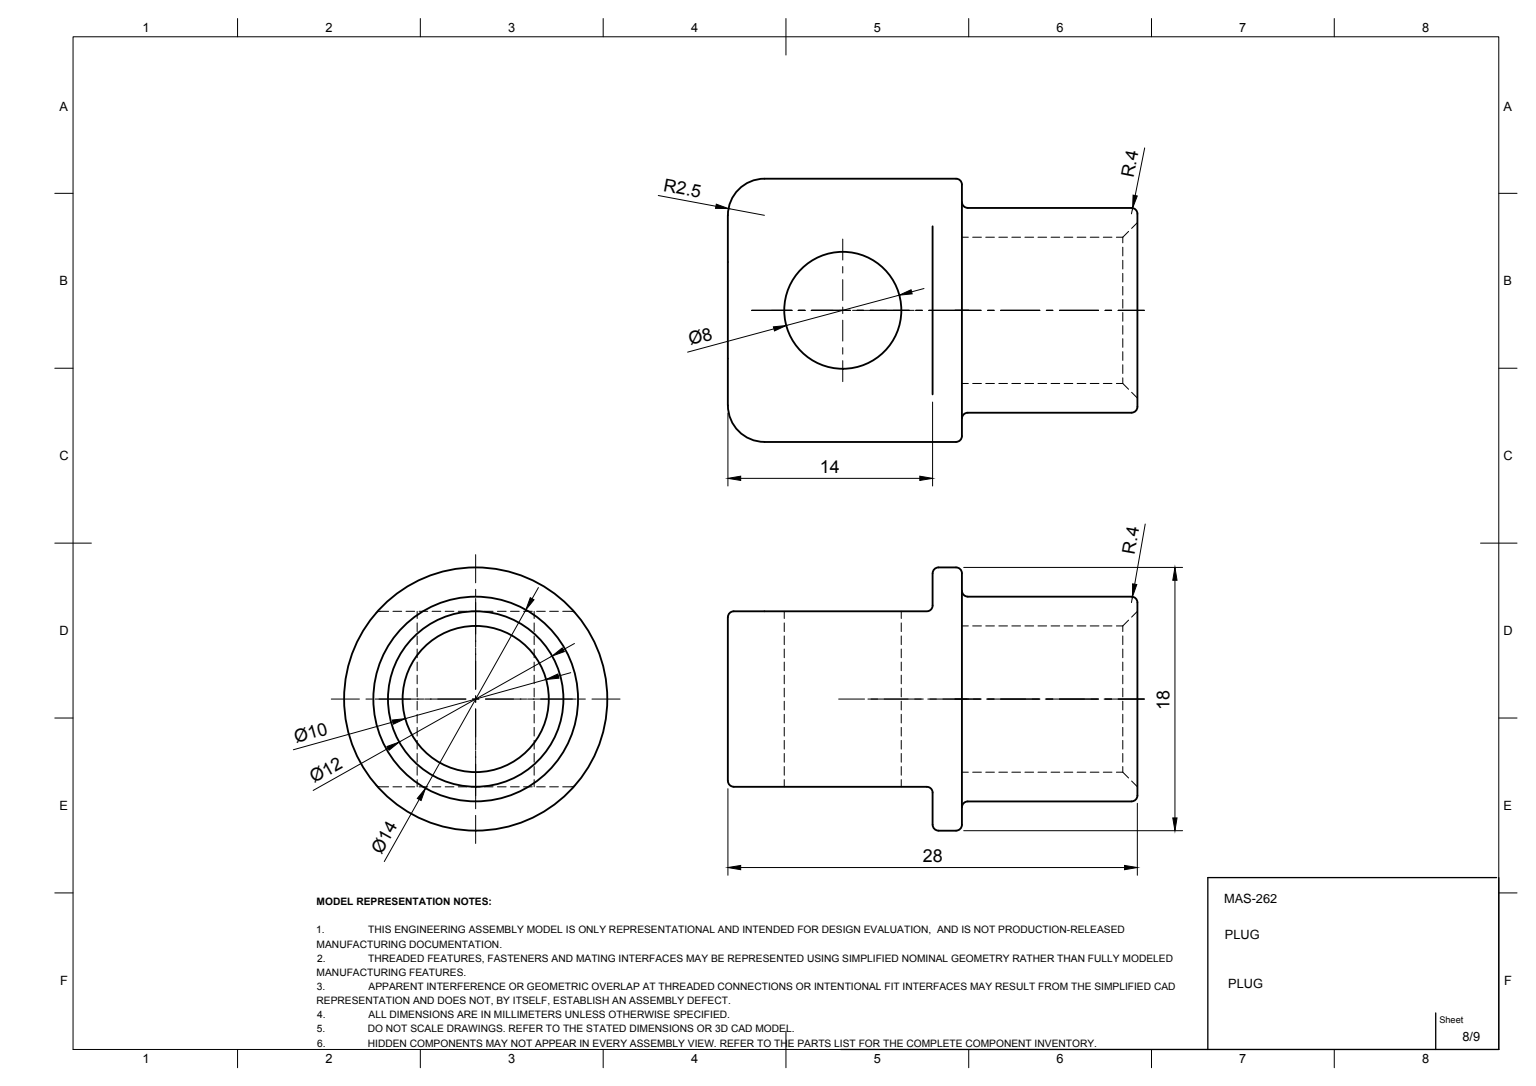
ISO-10303-21;
HEADER;
/* Generated by software containing ST-Developer
 * from STEP Tools, Inc. (www.steptools.com) 
 */

FILE_DESCRIPTION(
/* description */ (''),
/* implementation_level */ '2;1');

FILE_NAME(
/* name */ 'PLUG.step',
/* time_stamp */ '2026-10-07T02:13:48+06:00',
/* author */ (''),
/* organization */ (''),
/* preprocessor_version */ 'ST-DEVELOPER v20.2',
/* originating_system */ 'Autodesk Translation Framework v15.15.0.0',
/* authorisation */ '');

FILE_SCHEMA (('AUTOMOTIVE_DESIGN { 1 0 10303 214 3 1 1 }'));
ENDSEC;

DATA;
#10=MECHANICAL_DESIGN_GEOMETRIC_PRESENTATION_REPRESENTATION('',(#119),#17042);
#61=CONICAL_SURFACE('',#8902,5.5,0.785398163397441);
#76=B_SPLINE_SURFACE_WITH_KNOTS('',3,3,((#13698,#13699,#13700,#13701,#13702,
#13703),(#13704,#13705,#13706,#13707,#13708,#13709),(#13710,#13711,#13712,
#13713,#13714,#13715),(#13716,#13717,#13718,#13719,#13720,#13721),(#13722,
#13723,#13724,#13725,#13726,#13727)),.UNSPECIFIED.,.F.,.F.,.F.,(4,1,4),
(4,1,1,4),(0.,0.5,1.),(0.,0.0435664957825988,0.0599039317010734,0.0762413676195479),
 .UNSPECIFIED.);
#77=B_SPLINE_SURFACE_WITH_KNOTS('',3,3,((#13746,#13747,#13748,#13749,#13750,
#13751),(#13752,#13753,#13754,#13755,#13756,#13757),(#13758,#13759,#13760,
#13761,#13762,#13763),(#13764,#13765,#13766,#13767,#13768,#13769),(#13770,
#13771,#13772,#13773,#13774,#13775)),.UNSPECIFIED.,.F.,.F.,.F.,(4,1,4),
(4,1,1,4),(0.,0.5,1.),(0.,0.0163372895861103,0.0326745791722206,0.0762406847351813),
 .UNSPECIFIED.);
#78=B_SPLINE_SURFACE_WITH_KNOTS('',3,3,((#13800,#13801,#13802,#13803,#13804,
#13805),(#13806,#13807,#13808,#13809,#13810,#13811),(#13812,#13813,#13814,
#13815,#13816,#13817),(#13818,#13819,#13820,#13821,#13822,#13823),(#13824,
#13825,#13826,#13827,#13828,#13829)),.UNSPECIFIED.,.F.,.F.,.F.,(4,1,4),
(4,1,1,4),(0.,0.5,1.),(3.96177645312185E-16,0.061147749085529,0.0917216236282934,
0.214017121799351),.UNSPECIFIED.);
#79=B_SPLINE_SURFACE_WITH_KNOTS('',3,3,((#13851,#13852,#13853,#13854,#13855,
#13856),(#13857,#13858,#13859,#13860,#13861,#13862),(#13863,#13864,#13865,
#13866,#13867,#13868),(#13869,#13870,#13871,#13872,#13873,#13874),(#13875,
#13876,#13877,#13878,#13879,#13880)),.UNSPECIFIED.,.F.,.F.,.F.,(4,1,4),
(4,1,1,4),(0.,0.5,1.),(2.01858731750029E-18,0.0917257862177262,0.152876310362877,
0.214026834508028),.UNSPECIFIED.);
#80=B_SPLINE_SURFACE_WITH_KNOTS('',3,3,((#13926,#13927,#13928,#13929,#13930,
#13931),(#13932,#13933,#13934,#13935,#13936,#13937),(#13938,#13939,#13940,
#13941,#13942,#13943),(#13944,#13945,#13946,#13947,#13948,#13949),(#13950,
#13951,#13952,#13953,#13954,#13955)),.UNSPECIFIED.,.F.,.F.,.F.,(4,1,4),
(4,1,1,4),(0.,0.5,1.),(0.,0.0163372896496662,0.0326745792993324,0.0762406850317755),
 .UNSPECIFIED.);
#81=B_SPLINE_SURFACE_WITH_KNOTS('',3,3,((#13974,#13975,#13976,#13977,#13978,
#13979),(#13980,#13981,#13982,#13983,#13984,#13985),(#13986,#13987,#13988,
#13989,#13990,#13991),(#13992,#13993,#13994,#13995,#13996,#13997),(#13998,
#13999,#14000,#14001,#14002,#14003)),.UNSPECIFIED.,.F.,.F.,.F.,(4,1,4),
(4,1,1,4),(0.,0.5,1.),(7.01665201425609E-18,0.0435664948259872,0.0599039303857324,
0.0762413659454776),.UNSPECIFIED.);
#82=B_SPLINE_SURFACE_WITH_KNOTS('',3,3,((#14027,#14028,#14029,#14030,#14031,
#14032),(#14033,#14034,#14035,#14036,#14037,#14038),(#14039,#14040,#14041,
#14042,#14043,#14044),(#14045,#14046,#14047,#14048,#14049,#14050),(#14051,
#14052,#14053,#14054,#14055,#14056)),.UNSPECIFIED.,.F.,.F.,.F.,(4,1,4),
(4,1,1,4),(0.,0.5,1.),(6.74145042959343E-15,0.0611477488274177,0.0917216232411232,
0.214017120895945),.UNSPECIFIED.);
#83=B_SPLINE_SURFACE_WITH_KNOTS('',3,3,((#14069,#14070,#14071,#14072,#14073,
#14074),(#14075,#14076,#14077,#14078,#14079,#14080),(#14081,#14082,#14083,
#14084,#14085,#14086),(#14087,#14088,#14089,#14090,#14091,#14092),(#14093,
#14094,#14095,#14096,#14097,#14098)),.UNSPECIFIED.,.F.,.F.,.F.,(4,1,4),
(4,1,1,4),(0.,0.5,1.),(0.,0.0917257862177262,0.152876310362877,0.214026834508028),
 .UNSPECIFIED.);
#95=SHAPE_REPRESENTATION_RELATIONSHIP('SRR','None',#17091,#107);
#107=ADVANCED_BREP_SHAPE_REPRESENTATION('',(#131),#17035);
#119=STYLED_ITEM('',(#17154),#131);
#131=MANIFOLD_SOLID_BREP('Body1',#8120);
#164=FACE_BOUND('',#1281,.T.);
#165=FACE_BOUND('',#1294,.T.);
#166=FACE_BOUND('',#1299,.T.);
#167=FACE_BOUND('',#1304,.T.);
#226=TOROIDAL_SURFACE('',#8852,8.6,0.4);
#227=TOROIDAL_SURFACE('',#8859,6.5,2.5);
#228=TOROIDAL_SURFACE('',#8875,8.6,0.4);
#229=TOROIDAL_SURFACE('',#8885,6.5,2.5);
#230=TOROIDAL_SURFACE('',#8886,8.6,0.4);
#231=TOROIDAL_SURFACE('',#8891,7.4,0.4);
#232=TOROIDAL_SURFACE('',#8897,6.6,0.4);
#394=PLANE('',#8856);
#395=PLANE('',#8861);
#396=PLANE('',#8863);
#397=PLANE('',#8882);
#398=PLANE('',#8884);
#399=PLANE('',#8889);
#400=PLANE('',#8900);
#401=PLANE('',#8907);
#766=FACE_OUTER_BOUND('',#1269,.T.);
#767=FACE_OUTER_BOUND('',#1270,.T.);
#768=FACE_OUTER_BOUND('',#1271,.T.);
#769=FACE_OUTER_BOUND('',#1272,.T.);
#770=FACE_OUTER_BOUND('',#1273,.T.);
#771=FACE_OUTER_BOUND('',#1274,.T.);
#772=FACE_OUTER_BOUND('',#1275,.T.);
#773=FACE_OUTER_BOUND('',#1276,.T.);
#774=FACE_OUTER_BOUND('',#1277,.T.);
#775=FACE_OUTER_BOUND('',#1278,.T.);
#776=FACE_OUTER_BOUND('',#1279,.T.);
#777=FACE_OUTER_BOUND('',#1280,.T.);
#778=FACE_OUTER_BOUND('',#1282,.T.);
#779=FACE_OUTER_BOUND('',#1283,.T.);
#780=FACE_OUTER_BOUND('',#1284,.T.);
#781=FACE_OUTER_BOUND('',#1285,.T.);
#782=FACE_OUTER_BOUND('',#1286,.T.);
#783=FACE_OUTER_BOUND('',#1287,.T.);
#784=FACE_OUTER_BOUND('',#1288,.T.);
#785=FACE_OUTER_BOUND('',#1289,.T.);
#786=FACE_OUTER_BOUND('',#1290,.T.);
#787=FACE_OUTER_BOUND('',#1291,.T.);
#788=FACE_OUTER_BOUND('',#1292,.T.);
#789=FACE_OUTER_BOUND('',#1293,.T.);
#790=FACE_OUTER_BOUND('',#1295,.T.);
#791=FACE_OUTER_BOUND('',#1296,.T.);
#792=FACE_OUTER_BOUND('',#1297,.T.);
#793=FACE_OUTER_BOUND('',#1298,.T.);
#794=FACE_OUTER_BOUND('',#1300,.T.);
#795=FACE_OUTER_BOUND('',#1301,.T.);
#796=FACE_OUTER_BOUND('',#1302,.T.);
#797=FACE_OUTER_BOUND('',#1303,.T.);
#798=FACE_OUTER_BOUND('',#1305,.T.);
#799=FACE_OUTER_BOUND('',#1306,.T.);
#800=FACE_OUTER_BOUND('',#1307,.T.);
#801=FACE_OUTER_BOUND('',#1308,.T.);
#1269=EDGE_LOOP('',(#6539,#6540,#6541,#6542));
#1270=EDGE_LOOP('',(#6543,#6544,#6545,#6546));
#1271=EDGE_LOOP('',(#6547,#6548,#6549,#6550));
#1272=EDGE_LOOP('',(#6551,#6552,#6553,#6554));
#1273=EDGE_LOOP('',(#6555,#6556,#6557,#6558));
#1274=EDGE_LOOP('',(#6559,#6560,#6561,#6562));
#1275=EDGE_LOOP('',(#6563,#6564,#6565,#6566));
#1276=EDGE_LOOP('',(#6567,#6568,#6569,#6570));
#1277=EDGE_LOOP('',(#6571,#6572,#6573,#6574,#6575));
#1278=EDGE_LOOP('',(#6576,#6577,#6578,#6579));
#1279=EDGE_LOOP('',(#6580,#6581,#6582,#6583));
#1280=EDGE_LOOP('',(#6584,#6585,#6586,#6587,#6588,#6589));
#1281=EDGE_LOOP('',(#6590));
#1282=EDGE_LOOP('',(#6591,#6592));
#1283=EDGE_LOOP('',(#6593,#6594,#6595,#6596));
#1284=EDGE_LOOP('',(#6597,#6598,#6599,#6600));
#1285=EDGE_LOOP('',(#6601,#6602,#6603,#6604));
#1286=EDGE_LOOP('',(#6605,#6606,#6607,#6608));
#1287=EDGE_LOOP('',(#6609,#6610,#6611,#6612));
#1288=EDGE_LOOP('',(#6613,#6614,#6615,#6616));
#1289=EDGE_LOOP('',(#6617,#6618,#6619,#6620));
#1290=EDGE_LOOP('',(#6621,#6622,#6623,#6624));
#1291=EDGE_LOOP('',(#6625,#6626,#6627,#6628));
#1292=EDGE_LOOP('',(#6629,#6630,#6631,#6632,#6633,#6634,#6635,#6636,#6637,
#6638,#6639,#6640,#6641,#6642,#6643,#6644));
#1293=EDGE_LOOP('',(#6645,#6646,#6647,#6648,#6649,#6650));
#1294=EDGE_LOOP('',(#6651));
#1295=EDGE_LOOP('',(#6652,#6653));
#1296=EDGE_LOOP('',(#6654,#6655,#6656,#6657));
#1297=EDGE_LOOP('',(#6658,#6659,#6660,#6661));
#1298=EDGE_LOOP('',(#6662));
#1299=EDGE_LOOP('',(#6663));
#1300=EDGE_LOOP('',(#6664,#6665,#6666,#6667));
#1301=EDGE_LOOP('',(#6668,#6669,#6670,#6671,#6672));
#1302=EDGE_LOOP('',(#6673,#6674,#6675,#6676,#6677));
#1303=EDGE_LOOP('',(#6678));
#1304=EDGE_LOOP('',(#6679));
#1305=EDGE_LOOP('',(#6680,#6681,#6682,#6683));
#1306=EDGE_LOOP('',(#6684,#6685,#6686,#6687));
#1307=EDGE_LOOP('',(#6688,#6689,#6690,#6691));
#1308=EDGE_LOOP('',(#6692));
#1770=CIRCLE('',#8840,0.400000000000001);
#1771=CIRCLE('',#8841,0.399999999999991);
#1772=CIRCLE('',#8842,0.4);
#1773=CIRCLE('',#8843,0.400000000000001);
#1774=CIRCLE('',#8845,0.400000000000003);
#1775=CIRCLE('',#8846,0.4);
#1776=CIRCLE('',#8848,0.4);
#1777=CIRCLE('',#8849,0.4);
#1778=CIRCLE('',#8853,9.);
#1779=CIRCLE('',#8854,9.);
#1780=CIRCLE('',#8855,8.6);
#1781=CIRCLE('',#8857,6.5);
#1782=CIRCLE('',#8858,6.5);
#1783=CIRCLE('',#8860,9.);
#1784=CIRCLE('',#8862,4.);
#1785=CIRCLE('',#8864,0.4);
#1786=CIRCLE('',#8865,0.400000000000001);
#1787=CIRCLE('',#8866,0.400000000000001);
#1788=CIRCLE('',#8867,0.399999999999991);
#1789=CIRCLE('',#8869,0.4);
#1790=CIRCLE('',#8870,0.4);
#1791=CIRCLE('',#8872,0.399999999999999);
#1792=CIRCLE('',#8873,0.4);
#1793=CIRCLE('',#8876,9.);
#1794=CIRCLE('',#8877,8.6);
#1795=CIRCLE('',#8880,9.);
#1796=CIRCLE('',#8881,9.);
#1797=CIRCLE('',#8883,4.);
#1798=CIRCLE('',#8887,0.4);
#1799=CIRCLE('',#8888,8.6);
#1800=CIRCLE('',#8890,7.4);
#1801=CIRCLE('',#8892,7.);
#1802=CIRCLE('',#8893,0.4);
#1803=CIRCLE('',#8895,7.);
#1804=CIRCLE('',#8896,7.);
#1805=CIRCLE('',#8898,6.6);
#1806=CIRCLE('',#8899,0.4);
#1807=CIRCLE('',#8901,6.);
#1808=CIRCLE('',#8903,5.);
#1809=CIRCLE('',#8905,5.);
#1960=B_SPLINE_CURVE_WITH_KNOTS('',3,(#13730,#13731,#13732,#13733,#13734,
#13735),.UNSPECIFIED.,.F.,.F.,(4,1,1,4),(0.,0.0435664957825988,0.0599039317010734,
0.0762413676195479),.UNSPECIFIED.);
#1961=B_SPLINE_CURVE_WITH_KNOTS('',3,(#13739,#13740,#13741,#13742,#13743,
#13744),.UNSPECIFIED.,.F.,.F.,(4,1,1,4),(-0.0762413676195479,-0.0599039317010734,
-0.0435664957825988,0.),.UNSPECIFIED.);
#1962=B_SPLINE_CURVE_WITH_KNOTS('',3,(#13778,#13779,#13780,#13781,#13782,
#13783),.UNSPECIFIED.,.F.,.F.,(4,1,1,4),(-0.0762406847351813,-0.0326745791722206,
-0.0163372895861103,0.),.UNSPECIFIED.);
#1963=B_SPLINE_CURVE_WITH_KNOTS('',3,(#13787,#13788,#13789,#13790,#13791,
#13792),.UNSPECIFIED.,.F.,.F.,(4,1,1,4),(0.,0.0163372895861103,0.0326745791722206,
0.0762406847351813),.UNSPECIFIED.);
#1964=B_SPLINE_CURVE_WITH_KNOTS('',3,(#13833,#13834,#13835,#13836,#13837,
#13838),.UNSPECIFIED.,.F.,.F.,(4,1,1,4),(-0.214017121799351,-0.0917216236282934,
-0.061147749085529,-3.96177645312185E-16),.UNSPECIFIED.);
#1965=B_SPLINE_CURVE_WITH_KNOTS('',3,(#13839,#13840,#13841,#13842,#13843,
#13844),.UNSPECIFIED.,.F.,.F.,(4,1,1,4),(3.96177645312185E-16,0.061147749085529,
0.0917216236282934,0.214017121799351),.UNSPECIFIED.);
#1966=B_SPLINE_CURVE_WITH_KNOTS('',3,(#13884,#13885,#13886,#13887,#13888,
#13889),.UNSPECIFIED.,.F.,.F.,(4,1,1,4),(-0.214026834508028,-0.152876310362877,
-0.0917257862177262,-2.01858731750029E-18),.UNSPECIFIED.);
#1967=B_SPLINE_CURVE_WITH_KNOTS('',3,(#13890,#13891,#13892,#13893,#13894,
#13895),.UNSPECIFIED.,.F.,.F.,(4,1,1,4),(2.01858731750029E-18,0.0917257862177262,
0.152876310362877,0.214026834508028),.UNSPECIFIED.);
#1968=B_SPLINE_CURVE_WITH_KNOTS('',3,(#13916,#13917,#13918,#13919,#13920,
#13921),.UNSPECIFIED.,.F.,.F.,(4,1,1,4),(-0.214017120895945,-0.0917216232411232,
-0.0611477488274177,-6.74145042959343E-15),.UNSPECIFIED.);
#1969=B_SPLINE_CURVE_WITH_KNOTS('',3,(#13958,#13959,#13960,#13961,#13962,
#13963),.UNSPECIFIED.,.F.,.F.,(4,1,1,4),(-0.0762406850317755,-0.0326745792993324,
-0.0163372896496662,0.),.UNSPECIFIED.);
#1970=B_SPLINE_CURVE_WITH_KNOTS('',3,(#13967,#13968,#13969,#13970,#13971,
#13972),.UNSPECIFIED.,.F.,.F.,(4,1,1,4),(0.,0.0163372896496662,0.0326745792993324,
0.0762406850317755),.UNSPECIFIED.);
#1971=B_SPLINE_CURVE_WITH_KNOTS('',3,(#14006,#14007,#14008,#14009,#14010,
#14011),.UNSPECIFIED.,.F.,.F.,(4,1,1,4),(7.01665201425609E-18,0.0435664948259872,
0.0599039303857324,0.0762413659454776),.UNSPECIFIED.);
#1972=B_SPLINE_CURVE_WITH_KNOTS('',3,(#14015,#14016,#14017,#14018,#14019,
#14020),.UNSPECIFIED.,.F.,.F.,(4,1,1,4),(-0.0762413659454776,-0.0599039303857324,
-0.0435664948259872,-7.01665201425609E-18),.UNSPECIFIED.);
#1973=B_SPLINE_CURVE_WITH_KNOTS('',3,(#14059,#14060,#14061,#14062,#14063,
#14064),.UNSPECIFIED.,.F.,.F.,(4,1,1,4),(6.74145042959343E-15,0.0611477488274177,
0.0917216232411232,0.214017120895945),.UNSPECIFIED.);
#1974=B_SPLINE_CURVE_WITH_KNOTS('',3,(#14102,#14103,#14104,#14105,#14106,
#14107),.UNSPECIFIED.,.F.,.F.,(4,1,1,4),(-0.214026834508028,-0.152876310362877,
-0.0917257862177262,0.),.UNSPECIFIED.);
#1975=B_SPLINE_CURVE_WITH_KNOTS('',3,(#14108,#14109,#14110,#14111,#14112,
#14113),.UNSPECIFIED.,.F.,.F.,(4,1,1,4),(0.,0.0917257862177262,0.152876310362877,
0.214026834508028),.UNSPECIFIED.);
#2430=LINE('',#13798,#3008);
#2431=LINE('',#13799,#3009);
#2432=LINE('',#13849,#3010);
#2433=LINE('',#13850,#3011);
#2434=LINE('',#13897,#3012);
#2435=LINE('',#13898,#3013);
#2436=LINE('',#13900,#3014);
#2437=LINE('',#13901,#3015);
#2438=LINE('',#13911,#3016);
#2439=LINE('',#14025,#3017);
#2440=LINE('',#14026,#3018);
#2441=LINE('',#14068,#3019);
#2442=LINE('',#14115,#3020);
#2443=LINE('',#14116,#3021);
#2444=LINE('',#14121,#3022);
#2445=LINE('',#14122,#3023);
#2446=LINE('',#14126,#3024);
#2447=LINE('',#14148,#3025);
#2448=LINE('',#14159,#3026);
#2449=LINE('',#14163,#3027);
#2450=LINE('',#14166,#3028);
#3008=VECTOR('',#10831,20.);
#3009=VECTOR('',#10832,20.);
#3010=VECTOR('',#10839,20.);
#3011=VECTOR('',#10840,20.);
#3012=VECTOR('',#10845,20.);
#3013=VECTOR('',#10846,20.);
#3014=VECTOR('',#10849,20.);
#3015=VECTOR('',#10850,20.);
#3016=VECTOR('',#10863,20.);
#3017=VECTOR('',#10888,20.);
#3018=VECTOR('',#10889,20.);
#3019=VECTOR('',#10896,20.);
#3020=VECTOR('',#10901,20.);
#3021=VECTOR('',#10902,20.);
#3022=VECTOR('',#10911,20.);
#3023=VECTOR('',#10912,20.);
#3024=VECTOR('',#10917,9.);
#3025=VECTOR('',#10948,7.);
#3026=VECTOR('',#10963,5.5);
#3027=VECTOR('',#10968,5.);
#3028=VECTOR('',#10973,4.);
#3625=VERTEX_POINT('',#13728);
#3626=VERTEX_POINT('',#13729);
#3627=VERTEX_POINT('',#13736);
#3628=VERTEX_POINT('',#13738);
#3629=VERTEX_POINT('',#13776);
#3630=VERTEX_POINT('',#13777);
#3631=VERTEX_POINT('',#13784);
#3632=VERTEX_POINT('',#13786);
#3633=VERTEX_POINT('',#13795);
#3634=VERTEX_POINT('',#13796);
#3635=VERTEX_POINT('',#13830);
#3636=VERTEX_POINT('',#13831);
#3637=VERTEX_POINT('',#13846);
#3638=VERTEX_POINT('',#13847);
#3639=VERTEX_POINT('',#13881);
#3640=VERTEX_POINT('',#13882);
#3641=VERTEX_POINT('',#13903);
#3642=VERTEX_POINT('',#13908);
#3643=VERTEX_POINT('',#13910);
#3644=VERTEX_POINT('',#13914);
#3645=VERTEX_POINT('',#13923);
#3646=VERTEX_POINT('',#13956);
#3647=VERTEX_POINT('',#13957);
#3648=VERTEX_POINT('',#13964);
#3649=VERTEX_POINT('',#13966);
#3650=VERTEX_POINT('',#14004);
#3651=VERTEX_POINT('',#14005);
#3652=VERTEX_POINT('',#14012);
#3653=VERTEX_POINT('',#14014);
#3654=VERTEX_POINT('',#14023);
#3655=VERTEX_POINT('',#14057);
#3656=VERTEX_POINT('',#14066);
#3657=VERTEX_POINT('',#14099);
#3658=VERTEX_POINT('',#14100);
#3659=VERTEX_POINT('',#14125);
#3660=VERTEX_POINT('',#14129);
#3661=VERTEX_POINT('',#14134);
#3662=VERTEX_POINT('',#14138);
#3663=VERTEX_POINT('',#14141);
#3664=VERTEX_POINT('',#14145);
#3665=VERTEX_POINT('',#14146);
#3666=VERTEX_POINT('',#14151);
#3667=VERTEX_POINT('',#14155);
#3668=VERTEX_POINT('',#14158);
#3669=VERTEX_POINT('',#14162);
#4637=EDGE_CURVE('',#3625,#3626,#1960,.F.);
#4638=EDGE_CURVE('',#3627,#3625,#1770,.T.);
#4639=EDGE_CURVE('',#3627,#3628,#1961,.T.);
#4640=EDGE_CURVE('',#3626,#3628,#1771,.T.);
#4641=EDGE_CURVE('',#3629,#3630,#1962,.T.);
#4642=EDGE_CURVE('',#3631,#3630,#1772,.T.);
#4643=EDGE_CURVE('',#3632,#3631,#1963,.F.);
#4644=EDGE_CURVE('',#3629,#3632,#1773,.T.);
#4645=EDGE_CURVE('',#3633,#3634,#1774,.T.);
#4646=EDGE_CURVE('',#3634,#3627,#2430,.T.);
#4647=EDGE_CURVE('',#3625,#3633,#2431,.T.);
#4648=EDGE_CURVE('',#3635,#3636,#1775,.T.);
#4649=EDGE_CURVE('',#3636,#3634,#1964,.T.);
#4650=EDGE_CURVE('',#3633,#3635,#1965,.T.);
#4651=EDGE_CURVE('',#3637,#3638,#1776,.T.);
#4652=EDGE_CURVE('',#3638,#3636,#2432,.T.);
#4653=EDGE_CURVE('',#3635,#3637,#2433,.T.);
#4654=EDGE_CURVE('',#3639,#3640,#1777,.T.);
#4655=EDGE_CURVE('',#3640,#3638,#1966,.T.);
#4656=EDGE_CURVE('',#3637,#3639,#1967,.T.);
#4657=EDGE_CURVE('',#3630,#3640,#2434,.T.);
#4658=EDGE_CURVE('',#3639,#3631,#2435,.T.);
#4659=EDGE_CURVE('',#3631,#3625,#2436,.T.);
#4660=EDGE_CURVE('',#3626,#3632,#2437,.T.);
#4661=EDGE_CURVE('',#3628,#3641,#1778,.T.);
#4662=EDGE_CURVE('',#3641,#3629,#1779,.T.);
#4663=EDGE_CURVE('',#3632,#3626,#1780,.T.);
#4664=EDGE_CURVE('',#3642,#3638,#1781,.T.);
#4665=EDGE_CURVE('',#3643,#3642,#2438,.T.);
#4666=EDGE_CURVE('',#3636,#3643,#1782,.T.);
#4667=EDGE_CURVE('',#3640,#3644,#1783,.T.);
#4668=EDGE_CURVE('',#3642,#3644,#1968,.T.);
#4669=EDGE_CURVE('',#3645,#3645,#1784,.T.);
#4670=EDGE_CURVE('',#3646,#3647,#1969,.T.);
#4671=EDGE_CURVE('',#3648,#3647,#1785,.T.);
#4672=EDGE_CURVE('',#3649,#3648,#1970,.F.);
#4673=EDGE_CURVE('',#3646,#3649,#1786,.T.);
#4674=EDGE_CURVE('',#3650,#3651,#1971,.F.);
#4675=EDGE_CURVE('',#3652,#3650,#1787,.T.);
#4676=EDGE_CURVE('',#3652,#3653,#1972,.T.);
#4677=EDGE_CURVE('',#3651,#3653,#1788,.T.);
#4678=EDGE_CURVE('',#3654,#3644,#1789,.T.);
#4679=EDGE_CURVE('',#3644,#3652,#2439,.T.);
#4680=EDGE_CURVE('',#3650,#3654,#2440,.T.);
#4681=EDGE_CURVE('',#3655,#3642,#1790,.T.);
#4682=EDGE_CURVE('',#3654,#3655,#1973,.T.);
#4683=EDGE_CURVE('',#3656,#3643,#1791,.T.);
#4684=EDGE_CURVE('',#3655,#3656,#2441,.T.);
#4685=EDGE_CURVE('',#3657,#3658,#1792,.T.);
#4686=EDGE_CURVE('',#3658,#3643,#1974,.T.);
#4687=EDGE_CURVE('',#3656,#3657,#1975,.T.);
#4688=EDGE_CURVE('',#3647,#3658,#2442,.T.);
#4689=EDGE_CURVE('',#3657,#3648,#2443,.T.);
#4690=EDGE_CURVE('',#3653,#3646,#1793,.T.);
#4691=EDGE_CURVE('',#3649,#3651,#1794,.T.);
#4692=EDGE_CURVE('',#3648,#3650,#2444,.T.);
#4693=EDGE_CURVE('',#3651,#3649,#2445,.T.);
#4694=EDGE_CURVE('',#3658,#3634,#1795,.T.);
#4695=EDGE_CURVE('',#3641,#3659,#2446,.T.);
#4696=EDGE_CURVE('',#3659,#3659,#1796,.T.);
#4697=EDGE_CURVE('',#3660,#3660,#1797,.T.);
#4698=EDGE_CURVE('',#3659,#3661,#1798,.T.);
#4699=EDGE_CURVE('',#3661,#3661,#1799,.T.);
#4700=EDGE_CURVE('',#3662,#3662,#1800,.T.);
#4701=EDGE_CURVE('',#3663,#3663,#1801,.T.);
#4702=EDGE_CURVE('',#3663,#3662,#1802,.T.);
#4703=EDGE_CURVE('',#3664,#3665,#1803,.T.);
#4704=EDGE_CURVE('',#3664,#3663,#2447,.T.);
#4705=EDGE_CURVE('',#3665,#3664,#1804,.T.);
#4706=EDGE_CURVE('',#3666,#3666,#1805,.T.);
#4707=EDGE_CURVE('',#3666,#3665,#1806,.T.);
#4708=EDGE_CURVE('',#3667,#3667,#1807,.T.);
#4709=EDGE_CURVE('',#3667,#3668,#2448,.T.);
#4710=EDGE_CURVE('',#3668,#3668,#1808,.T.);
#4711=EDGE_CURVE('',#3668,#3669,#2449,.T.);
#4712=EDGE_CURVE('',#3669,#3669,#1809,.T.);
#4713=EDGE_CURVE('',#3645,#3660,#2450,.T.);
#6539=ORIENTED_EDGE('',*,*,#4637,.F.);
#6540=ORIENTED_EDGE('',*,*,#4638,.F.);
#6541=ORIENTED_EDGE('',*,*,#4639,.T.);
#6542=ORIENTED_EDGE('',*,*,#4640,.F.);
#6543=ORIENTED_EDGE('',*,*,#4641,.T.);
#6544=ORIENTED_EDGE('',*,*,#4642,.F.);
#6545=ORIENTED_EDGE('',*,*,#4643,.F.);
#6546=ORIENTED_EDGE('',*,*,#4644,.F.);
#6547=ORIENTED_EDGE('',*,*,#4645,.T.);
#6548=ORIENTED_EDGE('',*,*,#4646,.T.);
#6549=ORIENTED_EDGE('',*,*,#4638,.T.);
#6550=ORIENTED_EDGE('',*,*,#4647,.T.);
#6551=ORIENTED_EDGE('',*,*,#4648,.T.);
#6552=ORIENTED_EDGE('',*,*,#4649,.T.);
#6553=ORIENTED_EDGE('',*,*,#4645,.F.);
#6554=ORIENTED_EDGE('',*,*,#4650,.T.);
#6555=ORIENTED_EDGE('',*,*,#4651,.T.);
#6556=ORIENTED_EDGE('',*,*,#4652,.T.);
#6557=ORIENTED_EDGE('',*,*,#4648,.F.);
#6558=ORIENTED_EDGE('',*,*,#4653,.T.);
#6559=ORIENTED_EDGE('',*,*,#4654,.T.);
#6560=ORIENTED_EDGE('',*,*,#4655,.T.);
#6561=ORIENTED_EDGE('',*,*,#4651,.F.);
#6562=ORIENTED_EDGE('',*,*,#4656,.T.);
#6563=ORIENTED_EDGE('',*,*,#4642,.T.);
#6564=ORIENTED_EDGE('',*,*,#4657,.T.);
#6565=ORIENTED_EDGE('',*,*,#4654,.F.);
#6566=ORIENTED_EDGE('',*,*,#4658,.T.);
#6567=ORIENTED_EDGE('',*,*,#4643,.T.);
#6568=ORIENTED_EDGE('',*,*,#4659,.T.);
#6569=ORIENTED_EDGE('',*,*,#4637,.T.);
#6570=ORIENTED_EDGE('',*,*,#4660,.T.);
#6571=ORIENTED_EDGE('',*,*,#4640,.T.);
#6572=ORIENTED_EDGE('',*,*,#4661,.T.);
#6573=ORIENTED_EDGE('',*,*,#4662,.T.);
#6574=ORIENTED_EDGE('',*,*,#4644,.T.);
#6575=ORIENTED_EDGE('',*,*,#4663,.T.);
#6576=ORIENTED_EDGE('',*,*,#4652,.F.);
#6577=ORIENTED_EDGE('',*,*,#4664,.F.);
#6578=ORIENTED_EDGE('',*,*,#4665,.F.);
#6579=ORIENTED_EDGE('',*,*,#4666,.F.);
#6580=ORIENTED_EDGE('',*,*,#4655,.F.);
#6581=ORIENTED_EDGE('',*,*,#4667,.T.);
#6582=ORIENTED_EDGE('',*,*,#4668,.F.);
#6583=ORIENTED_EDGE('',*,*,#4664,.T.);
#6584=ORIENTED_EDGE('',*,*,#4647,.F.);
#6585=ORIENTED_EDGE('',*,*,#4659,.F.);
#6586=ORIENTED_EDGE('',*,*,#4658,.F.);
#6587=ORIENTED_EDGE('',*,*,#4656,.F.);
#6588=ORIENTED_EDGE('',*,*,#4653,.F.);
#6589=ORIENTED_EDGE('',*,*,#4650,.F.);
#6590=ORIENTED_EDGE('',*,*,#4669,.T.);
#6591=ORIENTED_EDGE('',*,*,#4660,.F.);
#6592=ORIENTED_EDGE('',*,*,#4663,.F.);
#6593=ORIENTED_EDGE('',*,*,#4670,.T.);
#6594=ORIENTED_EDGE('',*,*,#4671,.F.);
#6595=ORIENTED_EDGE('',*,*,#4672,.F.);
#6596=ORIENTED_EDGE('',*,*,#4673,.F.);
#6597=ORIENTED_EDGE('',*,*,#4674,.F.);
#6598=ORIENTED_EDGE('',*,*,#4675,.F.);
#6599=ORIENTED_EDGE('',*,*,#4676,.T.);
#6600=ORIENTED_EDGE('',*,*,#4677,.F.);
#6601=ORIENTED_EDGE('',*,*,#4678,.T.);
#6602=ORIENTED_EDGE('',*,*,#4679,.T.);
#6603=ORIENTED_EDGE('',*,*,#4675,.T.);
#6604=ORIENTED_EDGE('',*,*,#4680,.T.);
#6605=ORIENTED_EDGE('',*,*,#4681,.T.);
#6606=ORIENTED_EDGE('',*,*,#4668,.T.);
#6607=ORIENTED_EDGE('',*,*,#4678,.F.);
#6608=ORIENTED_EDGE('',*,*,#4682,.T.);
#6609=ORIENTED_EDGE('',*,*,#4683,.T.);
#6610=ORIENTED_EDGE('',*,*,#4665,.T.);
#6611=ORIENTED_EDGE('',*,*,#4681,.F.);
#6612=ORIENTED_EDGE('',*,*,#4684,.T.);
#6613=ORIENTED_EDGE('',*,*,#4685,.T.);
#6614=ORIENTED_EDGE('',*,*,#4686,.T.);
#6615=ORIENTED_EDGE('',*,*,#4683,.F.);
#6616=ORIENTED_EDGE('',*,*,#4687,.T.);
#6617=ORIENTED_EDGE('',*,*,#4671,.T.);
#6618=ORIENTED_EDGE('',*,*,#4688,.T.);
#6619=ORIENTED_EDGE('',*,*,#4685,.F.);
#6620=ORIENTED_EDGE('',*,*,#4689,.T.);
#6621=ORIENTED_EDGE('',*,*,#4677,.T.);
#6622=ORIENTED_EDGE('',*,*,#4690,.T.);
#6623=ORIENTED_EDGE('',*,*,#4673,.T.);
#6624=ORIENTED_EDGE('',*,*,#4691,.T.);
#6625=ORIENTED_EDGE('',*,*,#4672,.T.);
#6626=ORIENTED_EDGE('',*,*,#4692,.T.);
#6627=ORIENTED_EDGE('',*,*,#4674,.T.);
#6628=ORIENTED_EDGE('',*,*,#4693,.T.);
#6629=ORIENTED_EDGE('',*,*,#4646,.F.);
#6630=ORIENTED_EDGE('',*,*,#4694,.F.);
#6631=ORIENTED_EDGE('',*,*,#4688,.F.);
#6632=ORIENTED_EDGE('',*,*,#4670,.F.);
#6633=ORIENTED_EDGE('',*,*,#4690,.F.);
#6634=ORIENTED_EDGE('',*,*,#4676,.F.);
#6635=ORIENTED_EDGE('',*,*,#4679,.F.);
#6636=ORIENTED_EDGE('',*,*,#4667,.F.);
#6637=ORIENTED_EDGE('',*,*,#4657,.F.);
#6638=ORIENTED_EDGE('',*,*,#4641,.F.);
#6639=ORIENTED_EDGE('',*,*,#4662,.F.);
#6640=ORIENTED_EDGE('',*,*,#4695,.T.);
#6641=ORIENTED_EDGE('',*,*,#4696,.F.);
#6642=ORIENTED_EDGE('',*,*,#4695,.F.);
#6643=ORIENTED_EDGE('',*,*,#4661,.F.);
#6644=ORIENTED_EDGE('',*,*,#4639,.F.);
#6645=ORIENTED_EDGE('',*,*,#4680,.F.);
#6646=ORIENTED_EDGE('',*,*,#4692,.F.);
#6647=ORIENTED_EDGE('',*,*,#4689,.F.);
#6648=ORIENTED_EDGE('',*,*,#4687,.F.);
#6649=ORIENTED_EDGE('',*,*,#4684,.F.);
#6650=ORIENTED_EDGE('',*,*,#4682,.F.);
#6651=ORIENTED_EDGE('',*,*,#4697,.T.);
#6652=ORIENTED_EDGE('',*,*,#4691,.F.);
#6653=ORIENTED_EDGE('',*,*,#4693,.F.);
#6654=ORIENTED_EDGE('',*,*,#4649,.F.);
#6655=ORIENTED_EDGE('',*,*,#4666,.T.);
#6656=ORIENTED_EDGE('',*,*,#4686,.F.);
#6657=ORIENTED_EDGE('',*,*,#4694,.T.);
#6658=ORIENTED_EDGE('',*,*,#4696,.T.);
#6659=ORIENTED_EDGE('',*,*,#4698,.T.);
#6660=ORIENTED_EDGE('',*,*,#4699,.T.);
#6661=ORIENTED_EDGE('',*,*,#4698,.F.);
#6662=ORIENTED_EDGE('',*,*,#4699,.F.);
#6663=ORIENTED_EDGE('',*,*,#4700,.F.);
#6664=ORIENTED_EDGE('',*,*,#4701,.T.);
#6665=ORIENTED_EDGE('',*,*,#4702,.T.);
#6666=ORIENTED_EDGE('',*,*,#4700,.T.);
#6667=ORIENTED_EDGE('',*,*,#4702,.F.);
#6668=ORIENTED_EDGE('',*,*,#4703,.F.);
#6669=ORIENTED_EDGE('',*,*,#4704,.T.);
#6670=ORIENTED_EDGE('',*,*,#4701,.F.);
#6671=ORIENTED_EDGE('',*,*,#4704,.F.);
#6672=ORIENTED_EDGE('',*,*,#4705,.F.);
#6673=ORIENTED_EDGE('',*,*,#4706,.T.);
#6674=ORIENTED_EDGE('',*,*,#4707,.T.);
#6675=ORIENTED_EDGE('',*,*,#4705,.T.);
#6676=ORIENTED_EDGE('',*,*,#4703,.T.);
#6677=ORIENTED_EDGE('',*,*,#4707,.F.);
#6678=ORIENTED_EDGE('',*,*,#4706,.F.);
#6679=ORIENTED_EDGE('',*,*,#4708,.F.);
#6680=ORIENTED_EDGE('',*,*,#4708,.T.);
#6681=ORIENTED_EDGE('',*,*,#4709,.T.);
#6682=ORIENTED_EDGE('',*,*,#4710,.T.);
#6683=ORIENTED_EDGE('',*,*,#4709,.F.);
#6684=ORIENTED_EDGE('',*,*,#4710,.F.);
#6685=ORIENTED_EDGE('',*,*,#4711,.T.);
#6686=ORIENTED_EDGE('',*,*,#4712,.F.);
#6687=ORIENTED_EDGE('',*,*,#4711,.F.);
#6688=ORIENTED_EDGE('',*,*,#4669,.F.);
#6689=ORIENTED_EDGE('',*,*,#4713,.T.);
#6690=ORIENTED_EDGE('',*,*,#4697,.F.);
#6691=ORIENTED_EDGE('',*,*,#4713,.F.);
#6692=ORIENTED_EDGE('',*,*,#4712,.T.);
#7571=CYLINDRICAL_SURFACE('',#8844,0.4);
#7572=CYLINDRICAL_SURFACE('',#8847,0.4);
#7573=CYLINDRICAL_SURFACE('',#8850,0.4);
#7574=CYLINDRICAL_SURFACE('',#8851,0.4);
#7575=CYLINDRICAL_SURFACE('',#8868,0.4);
#7576=CYLINDRICAL_SURFACE('',#8871,0.4);
#7577=CYLINDRICAL_SURFACE('',#8874,0.4);
#7578=CYLINDRICAL_SURFACE('',#8878,0.4);
#7579=CYLINDRICAL_SURFACE('',#8879,9.);
#7580=CYLINDRICAL_SURFACE('',#8894,7.);
#7581=CYLINDRICAL_SURFACE('',#8904,5.);
#7582=CYLINDRICAL_SURFACE('',#8906,4.);
#7928=ADVANCED_FACE('',(#766),#76,.F.);
#7929=ADVANCED_FACE('',(#767),#77,.F.);
#7930=ADVANCED_FACE('',(#768),#7571,.T.);
#7931=ADVANCED_FACE('',(#769),#78,.F.);
#7932=ADVANCED_FACE('',(#770),#7572,.T.);
#7933=ADVANCED_FACE('',(#771),#79,.F.);
#7934=ADVANCED_FACE('',(#772),#7573,.T.);
#7935=ADVANCED_FACE('',(#773),#7574,.F.);
#7936=ADVANCED_FACE('',(#774),#226,.T.);
#7937=ADVANCED_FACE('',(#775),#394,.T.);
#7938=ADVANCED_FACE('',(#776),#227,.T.);
#7939=ADVANCED_FACE('',(#777,#164),#395,.F.);
#7940=ADVANCED_FACE('',(#778),#396,.T.);
#7941=ADVANCED_FACE('',(#779),#80,.F.);
#7942=ADVANCED_FACE('',(#780),#81,.F.);
#7943=ADVANCED_FACE('',(#781),#7575,.T.);
#7944=ADVANCED_FACE('',(#782),#82,.F.);
#7945=ADVANCED_FACE('',(#783),#7576,.T.);
#7946=ADVANCED_FACE('',(#784),#83,.F.);
#7947=ADVANCED_FACE('',(#785),#7577,.T.);
#7948=ADVANCED_FACE('',(#786),#228,.T.);
#7949=ADVANCED_FACE('',(#787),#7578,.F.);
#7950=ADVANCED_FACE('',(#788),#7579,.T.);
#7951=ADVANCED_FACE('',(#789,#165),#397,.F.);
#7952=ADVANCED_FACE('',(#790),#398,.T.);
#7953=ADVANCED_FACE('',(#791),#229,.T.);
#7954=ADVANCED_FACE('',(#792),#230,.T.);
#7955=ADVANCED_FACE('',(#793,#166),#399,.F.);
#7956=ADVANCED_FACE('',(#794),#231,.F.);
#7957=ADVANCED_FACE('',(#795),#7580,.T.);
#7958=ADVANCED_FACE('',(#796),#232,.T.);
#7959=ADVANCED_FACE('',(#797,#167),#400,.F.);
#7960=ADVANCED_FACE('',(#798),#61,.F.);
#7961=ADVANCED_FACE('',(#799),#7581,.F.);
#7962=ADVANCED_FACE('',(#800),#7582,.F.);
#7963=ADVANCED_FACE('',(#801),#401,.F.);
#8120=CLOSED_SHELL('',(#7928,#7929,#7930,#7931,#7932,#7933,#7934,#7935,
#7936,#7937,#7938,#7939,#7940,#7941,#7942,#7943,#7944,#7945,#7946,#7947,
#7948,#7949,#7950,#7951,#7952,#7953,#7954,#7955,#7956,#7957,#7958,#7959,
#7960,#7961,#7962,#7963));
#8839=AXIS2_PLACEMENT_3D('',#13697,#10817,#10818);
#8840=AXIS2_PLACEMENT_3D('',#13737,#10819,#10820);
#8841=AXIS2_PLACEMENT_3D('',#13745,#10821,#10822);
#8842=AXIS2_PLACEMENT_3D('',#13785,#10823,#10824);
#8843=AXIS2_PLACEMENT_3D('',#13793,#10825,#10826);
#8844=AXIS2_PLACEMENT_3D('',#13794,#10827,#10828);
#8845=AXIS2_PLACEMENT_3D('',#13797,#10829,#10830);
#8846=AXIS2_PLACEMENT_3D('',#13832,#10833,#10834);
#8847=AXIS2_PLACEMENT_3D('',#13845,#10835,#10836);
#8848=AXIS2_PLACEMENT_3D('',#13848,#10837,#10838);
#8849=AXIS2_PLACEMENT_3D('',#13883,#10841,#10842);
#8850=AXIS2_PLACEMENT_3D('',#13896,#10843,#10844);
#8851=AXIS2_PLACEMENT_3D('',#13899,#10847,#10848);
#8852=AXIS2_PLACEMENT_3D('',#13902,#10851,#10852);
#8853=AXIS2_PLACEMENT_3D('',#13904,#10853,#10854);
#8854=AXIS2_PLACEMENT_3D('',#13905,#10855,#10856);
#8855=AXIS2_PLACEMENT_3D('',#13906,#10857,#10858);
#8856=AXIS2_PLACEMENT_3D('',#13907,#10859,#10860);
#8857=AXIS2_PLACEMENT_3D('',#13909,#10861,#10862);
#8858=AXIS2_PLACEMENT_3D('',#13912,#10864,#10865);
#8859=AXIS2_PLACEMENT_3D('',#13913,#10866,#10867);
#8860=AXIS2_PLACEMENT_3D('',#13915,#10868,#10869);
#8861=AXIS2_PLACEMENT_3D('',#13922,#10870,#10871);
#8862=AXIS2_PLACEMENT_3D('',#13924,#10872,#10873);
#8863=AXIS2_PLACEMENT_3D('',#13925,#10874,#10875);
#8864=AXIS2_PLACEMENT_3D('',#13965,#10876,#10877);
#8865=AXIS2_PLACEMENT_3D('',#13973,#10878,#10879);
#8866=AXIS2_PLACEMENT_3D('',#14013,#10880,#10881);
#8867=AXIS2_PLACEMENT_3D('',#14021,#10882,#10883);
#8868=AXIS2_PLACEMENT_3D('',#14022,#10884,#10885);
#8869=AXIS2_PLACEMENT_3D('',#14024,#10886,#10887);
#8870=AXIS2_PLACEMENT_3D('',#14058,#10890,#10891);
#8871=AXIS2_PLACEMENT_3D('',#14065,#10892,#10893);
#8872=AXIS2_PLACEMENT_3D('',#14067,#10894,#10895);
#8873=AXIS2_PLACEMENT_3D('',#14101,#10897,#10898);
#8874=AXIS2_PLACEMENT_3D('',#14114,#10899,#10900);
#8875=AXIS2_PLACEMENT_3D('',#14117,#10903,#10904);
#8876=AXIS2_PLACEMENT_3D('',#14118,#10905,#10906);
#8877=AXIS2_PLACEMENT_3D('',#14119,#10907,#10908);
#8878=AXIS2_PLACEMENT_3D('',#14120,#10909,#10910);
#8879=AXIS2_PLACEMENT_3D('',#14123,#10913,#10914);
#8880=AXIS2_PLACEMENT_3D('',#14124,#10915,#10916);
#8881=AXIS2_PLACEMENT_3D('',#14127,#10918,#10919);
#8882=AXIS2_PLACEMENT_3D('',#14128,#10920,#10921);
#8883=AXIS2_PLACEMENT_3D('',#14130,#10922,#10923);
#8884=AXIS2_PLACEMENT_3D('',#14131,#10924,#10925);
#8885=AXIS2_PLACEMENT_3D('',#14132,#10926,#10927);
#8886=AXIS2_PLACEMENT_3D('',#14133,#10928,#10929);
#8887=AXIS2_PLACEMENT_3D('',#14135,#10930,#10931);
#8888=AXIS2_PLACEMENT_3D('',#14136,#10932,#10933);
#8889=AXIS2_PLACEMENT_3D('',#14137,#10934,#10935);
#8890=AXIS2_PLACEMENT_3D('',#14139,#10936,#10937);
#8891=AXIS2_PLACEMENT_3D('',#14140,#10938,#10939);
#8892=AXIS2_PLACEMENT_3D('',#14142,#10940,#10941);
#8893=AXIS2_PLACEMENT_3D('',#14143,#10942,#10943);
#8894=AXIS2_PLACEMENT_3D('',#14144,#10944,#10945);
#8895=AXIS2_PLACEMENT_3D('',#14147,#10946,#10947);
#8896=AXIS2_PLACEMENT_3D('',#14149,#10949,#10950);
#8897=AXIS2_PLACEMENT_3D('',#14150,#10951,#10952);
#8898=AXIS2_PLACEMENT_3D('',#14152,#10953,#10954);
#8899=AXIS2_PLACEMENT_3D('',#14153,#10955,#10956);
#8900=AXIS2_PLACEMENT_3D('',#14154,#10957,#10958);
#8901=AXIS2_PLACEMENT_3D('',#14156,#10959,#10960);
#8902=AXIS2_PLACEMENT_3D('',#14157,#10961,#10962);
#8903=AXIS2_PLACEMENT_3D('',#14160,#10964,#10965);
#8904=AXIS2_PLACEMENT_3D('',#14161,#10966,#10967);
#8905=AXIS2_PLACEMENT_3D('',#14164,#10969,#10970);
#8906=AXIS2_PLACEMENT_3D('',#14165,#10971,#10972);
#8907=AXIS2_PLACEMENT_3D('',#14167,#10974,#10975);
#10817=DIRECTION('axis',(0.,0.,1.));
#10818=DIRECTION('refdir',(1.,0.,0.));
#10819=DIRECTION('center_axis',(0.,0.,1.));
#10820=DIRECTION('ref_axis',(-0.651162790697674,0.758938087073522,0.));
#10821=DIRECTION('center_axis',(-0.667972400760236,-0.744186046511628,0.));
#10822=DIRECTION('ref_axis',(0.,0.,1.));
#10823=DIRECTION('center_axis',(0.,0.,1.));
#10824=DIRECTION('ref_axis',(-1.,0.,0.));
#10825=DIRECTION('center_axis',(-0.667972400760235,0.744186046511629,5.98505826505541E-15));
#10826=DIRECTION('ref_axis',(-0.744186046511629,-0.667972400760235,0.));
#10827=DIRECTION('center_axis',(0.,0.,1.));
#10828=DIRECTION('ref_axis',(-0.908615097469131,0.417634534792277,0.));
#10829=DIRECTION('center_axis',(0.,0.,-1.));
#10830=DIRECTION('ref_axis',(-1.,0.,0.));
#10831=DIRECTION('',(0.,0.,-1.));
#10832=DIRECTION('',(0.,0.,1.));
#10833=DIRECTION('center_axis',(0.,1.,1.80411241501592E-14));
#10834=DIRECTION('ref_axis',(-1.,0.,0.));
#10835=DIRECTION('center_axis',(-2.01858731750028E-16,-1.,0.));
#10836=DIRECTION('ref_axis',(-0.707106781186618,0.,0.707106781186477));
#10837=DIRECTION('center_axis',(0.,1.,1.38777878078148E-15));
#10838=DIRECTION('ref_axis',(-1.,0.,0.));
#10839=DIRECTION('',(2.01858731750028E-16,1.,0.));
#10840=DIRECTION('',(-2.01858731750028E-16,-1.,0.));
#10841=DIRECTION('center_axis',(0.,0.,1.));
#10842=DIRECTION('ref_axis',(-1.,-2.77555756156289E-15,0.));
#10843=DIRECTION('center_axis',(0.,0.,-1.));
#10844=DIRECTION('ref_axis',(-0.90861509746913,-0.417634534792279,0.));
#10845=DIRECTION('',(0.,0.,1.));
#10846=DIRECTION('',(0.,0.,-1.));
#10847=DIRECTION('center_axis',(-2.01858731750028E-16,-1.,0.));
#10848=DIRECTION('ref_axis',(0.707106781186493,0.,-0.707106781186602));
#10849=DIRECTION('',(2.01858731750028E-16,1.,0.));
#10850=DIRECTION('',(-2.01858731750028E-16,-1.,0.));
#10851=DIRECTION('center_axis',(0.,0.,-1.));
#10852=DIRECTION('ref_axis',(-1.,0.,0.));
#10853=DIRECTION('center_axis',(0.,0.,1.));
#10854=DIRECTION('ref_axis',(-1.,-1.22464679914735E-16,0.));
#10855=DIRECTION('center_axis',(0.,0.,1.));
#10856=DIRECTION('ref_axis',(-1.,-1.22464679914735E-16,0.));
#10857=DIRECTION('center_axis',(0.,0.,-1.));
#10858=DIRECTION('ref_axis',(-1.,-1.22464679914735E-16,0.));
#10859=DIRECTION('center_axis',(0.,0.,1.));
#10860=DIRECTION('ref_axis',(1.,0.,0.));
#10861=DIRECTION('center_axis',(0.,0.,-1.));
#10862=DIRECTION('ref_axis',(6.12323399573677E-17,-1.,0.));
#10863=DIRECTION('',(-1.51394048812521E-16,-1.,0.));
#10864=DIRECTION('center_axis',(0.,0.,-1.));
#10865=DIRECTION('ref_axis',(5.0532154980743E-16,1.,0.));
#10866=DIRECTION('center_axis',(0.,0.,1.));
#10867=DIRECTION('ref_axis',(1.,0.,0.));
#10868=DIRECTION('center_axis',(0.,0.,1.));
#10869=DIRECTION('ref_axis',(6.12323399573677E-17,-1.,0.));
#10870=DIRECTION('center_axis',(1.,-2.01858731750028E-16,0.));
#10871=DIRECTION('ref_axis',(-2.01858731750028E-16,-1.,0.));
#10872=DIRECTION('center_axis',(1.,-2.01858731750028E-16,0.));
#10873=DIRECTION('ref_axis',(0.,-1.,0.));
#10874=DIRECTION('center_axis',(0.,0.,1.));
#10875=DIRECTION('ref_axis',(-1.,0.,0.));
#10876=DIRECTION('center_axis',(0.,0.,1.));
#10877=DIRECTION('ref_axis',(1.,0.,0.));
#10878=DIRECTION('center_axis',(0.667972400760235,-0.744186046511629,-2.06553120860499E-15));
#10879=DIRECTION('ref_axis',(0.744186046511629,0.667972400760235,0.));
#10880=DIRECTION('center_axis',(0.,0.,1.));
#10881=DIRECTION('ref_axis',(0.651162790697674,-0.758938087073522,0.));
#10882=DIRECTION('center_axis',(0.667972400760231,0.744186046511633,0.));
#10883=DIRECTION('ref_axis',(0.,0.,1.));
#10884=DIRECTION('center_axis',(0.,0.,1.));
#10885=DIRECTION('ref_axis',(0.90861509746913,-0.417634534792279,0.));
#10886=DIRECTION('center_axis',(0.,0.,-1.));
#10887=DIRECTION('ref_axis',(1.,0.,0.));
#10888=DIRECTION('',(0.,0.,-1.));
#10889=DIRECTION('',(0.,0.,1.));
#10890=DIRECTION('center_axis',(0.,-1.,2.9143354396411E-14));
#10891=DIRECTION('ref_axis',(1.,0.,0.));
#10892=DIRECTION('center_axis',(1.51394048812521E-16,1.,0.));
#10893=DIRECTION('ref_axis',(0.707106781186618,0.,0.707106781186477));
#10894=DIRECTION('center_axis',(0.,-1.,0.));
#10895=DIRECTION('ref_axis',(1.,0.,0.));
#10896=DIRECTION('',(1.51394048812521E-16,1.,0.));
#10897=DIRECTION('center_axis',(0.,0.,1.));
#10898=DIRECTION('ref_axis',(1.,2.77555756156289E-15,0.));
#10899=DIRECTION('center_axis',(0.,0.,-1.));
#10900=DIRECTION('ref_axis',(0.90861509746913,0.417634534792279,0.));
#10901=DIRECTION('',(0.,0.,1.));
#10902=DIRECTION('',(0.,0.,-1.));
#10903=DIRECTION('center_axis',(0.,0.,-1.));
#10904=DIRECTION('ref_axis',(1.,-9.86864910777917E-17,0.));
#10905=DIRECTION('center_axis',(0.,0.,1.));
#10906=DIRECTION('ref_axis',(1.,-5.55111512312578E-17,0.));
#10907=DIRECTION('center_axis',(0.,0.,-1.));
#10908=DIRECTION('ref_axis',(1.,-5.55111512312578E-17,0.));
#10909=DIRECTION('center_axis',(1.51394048812521E-16,1.,0.));
#10910=DIRECTION('ref_axis',(-0.707106781186493,0.,-0.707106781186602));
#10911=DIRECTION('',(-1.51394048812521E-16,-1.,0.));
#10912=DIRECTION('',(1.51394048812521E-16,1.,0.));
#10913=DIRECTION('center_axis',(0.,0.,1.));
#10914=DIRECTION('ref_axis',(1.,0.,0.));
#10915=DIRECTION('center_axis',(0.,0.,1.));
#10916=DIRECTION('ref_axis',(5.0532154980743E-16,1.,0.));
#10917=DIRECTION('',(0.,0.,-1.));
#10918=DIRECTION('center_axis',(0.,0.,-1.));
#10919=DIRECTION('ref_axis',(1.,0.,0.));
#10920=DIRECTION('center_axis',(-1.,1.51394048812521E-16,0.));
#10921=DIRECTION('ref_axis',(1.51394048812521E-16,1.,0.));
#10922=DIRECTION('center_axis',(-1.,1.51394048812521E-16,0.));
#10923=DIRECTION('ref_axis',(0.,-1.,0.));
#10924=DIRECTION('center_axis',(0.,0.,1.));
#10925=DIRECTION('ref_axis',(-1.,0.,0.));
#10926=DIRECTION('center_axis',(0.,0.,1.));
#10927=DIRECTION('ref_axis',(1.,0.,0.));
#10928=DIRECTION('center_axis',(0.,0.,1.));
#10929=DIRECTION('ref_axis',(1.,0.,0.));
#10930=DIRECTION('center_axis',(1.2335811384724E-16,-1.,0.));
#10931=DIRECTION('ref_axis',(-1.,-1.2335811384724E-16,0.));
#10932=DIRECTION('center_axis',(0.,0.,1.));
#10933=DIRECTION('ref_axis',(1.,0.,0.));
#10934=DIRECTION('center_axis',(0.,0.,1.));
#10935=DIRECTION('ref_axis',(1.,0.,0.));
#10936=DIRECTION('center_axis',(0.,0.,-1.));
#10937=DIRECTION('ref_axis',(1.,0.,0.));
#10938=DIRECTION('center_axis',(0.,0.,1.));
#10939=DIRECTION('ref_axis',(1.,0.,0.));
#10940=DIRECTION('center_axis',(0.,0.,1.));
#10941=DIRECTION('ref_axis',(1.,0.,0.));
#10942=DIRECTION('center_axis',(1.42336285208353E-16,-1.,0.));
#10943=DIRECTION('ref_axis',(-1.,-1.42336285208353E-16,0.));
#10944=DIRECTION('center_axis',(0.,0.,-1.));
#10945=DIRECTION('ref_axis',(1.,0.,0.));
#10946=DIRECTION('center_axis',(0.,0.,-1.));
#10947=DIRECTION('ref_axis',(1.,0.,0.));
#10948=DIRECTION('',(0.,0.,1.));
#10949=DIRECTION('center_axis',(0.,0.,-1.));
#10950=DIRECTION('ref_axis',(1.,0.,0.));
#10951=DIRECTION('center_axis',(0.,0.,-1.));
#10952=DIRECTION('ref_axis',(-1.,0.,0.));
#10953=DIRECTION('center_axis',(0.,0.,1.));
#10954=DIRECTION('ref_axis',(1.,0.,0.));
#10955=DIRECTION('center_axis',(-1.58603289232165E-16,-1.,0.));
#10956=DIRECTION('ref_axis',(1.,-1.58603289232165E-16,0.));
#10957=DIRECTION('center_axis',(0.,0.,1.));
#10958=DIRECTION('ref_axis',(1.,0.,0.));
#10959=DIRECTION('center_axis',(0.,0.,-1.));
#10960=DIRECTION('ref_axis',(1.,0.,0.));
#10961=DIRECTION('center_axis',(0.,0.,-1.));
#10962=DIRECTION('ref_axis',(1.,0.,0.));
#10963=DIRECTION('',(0.707106781186542,-8.65956056235487E-17,0.707106781186553));
#10964=DIRECTION('center_axis',(0.,0.,1.));
#10965=DIRECTION('ref_axis',(1.,0.,0.));
#10966=DIRECTION('center_axis',(0.,0.,-1.));
#10967=DIRECTION('ref_axis',(1.,0.,0.));
#10968=DIRECTION('',(0.,0.,1.));
#10969=DIRECTION('center_axis',(0.,0.,-1.));
#10970=DIRECTION('ref_axis',(1.,0.,0.));
#10971=DIRECTION('center_axis',(1.,0.,0.));
#10972=DIRECTION('ref_axis',(0.,-1.,0.));
#10973=DIRECTION('',(1.,0.,0.));
#10974=DIRECTION('center_axis',(0.,0.,1.));
#10975=DIRECTION('ref_axis',(1.,0.,0.));
#13697=CARTESIAN_POINT('',(0.,0.,0.));
#13698=CARTESIAN_POINT('Ctrl Pts',(-12.9,12.1763356291059,464.946209595194));
#13699=CARTESIAN_POINT('Ctrl Pts',(-12.8029959440646,12.3924794841513,464.946209595194));
#13700=CARTESIAN_POINT('Ctrl Pts',(-12.6563710262499,12.683434963611,464.993269980864));
#13701=CARTESIAN_POINT('Ctrl Pts',(-12.5230694771437,12.9192723440419,465.183424929997));
#13702=CARTESIAN_POINT('Ctrl Pts',(-12.5,12.9586405314001,465.291751475466));
#13703=CARTESIAN_POINT('Ctrl Pts',(-12.5,12.9586405314001,465.346209595194));
#13704=CARTESIAN_POINT('Ctrl Pts',(-12.9779309805542,12.2462855353402,464.946209595194));
#13705=CARTESIAN_POINT('Ctrl Pts',(-12.8697226228569,12.4569505293086,464.926883433363));
#13706=CARTESIAN_POINT('Ctrl Pts',(-12.6938330928061,12.7438388264629,464.958568912738));
#13707=CARTESIAN_POINT('Ctrl Pts',(-12.5288182589974,12.9770526459975,465.163348776432));
#13708=CARTESIAN_POINT('Ctrl Pts',(-12.5,13.0160859158435,465.285050299185));
#13709=CARTESIAN_POINT('Ctrl Pts',(-12.5,13.0160859158435,465.346209595194));
#13710=CARTESIAN_POINT('Ctrl Pts',(-13.1330572932533,12.3855250386881,464.859380333003));
#13711=CARTESIAN_POINT('Ctrl Pts',(-12.9815601460676,12.5859161586474,464.824024352416));
#13712=CARTESIAN_POINT('Ctrl Pts',(-12.7386227137214,12.8645013145008,464.854838097387));
#13713=CARTESIAN_POINT('Ctrl Pts',(-12.5140044782818,13.092657901597,465.113239520754));
#13714=CARTESIAN_POINT('Ctrl Pts',(-12.4748408805091,13.1309318538629,465.268197789592));
#13715=CARTESIAN_POINT('Ctrl Pts',(-12.4748408805091,13.1309318538629,465.346209595194));
#13716=CARTESIAN_POINT('Ctrl Pts',(-13.1976744186047,12.44352458941,464.650929350314));
#13717=CARTESIAN_POINT('Ctrl Pts',(-13.0056838626847,12.6568334505882,464.638779692075));
#13718=CARTESIAN_POINT('Ctrl Pts',(-12.7145954604713,12.9482471139396,464.711880095389));
#13719=CARTESIAN_POINT('Ctrl Pts',(-12.4497756270675,13.1850735534976,465.051466709479));
#13720=CARTESIAN_POINT('Ctrl Pts',(-12.4040626064597,13.2248094693827,465.247599949711));
#13721=CARTESIAN_POINT('Ctrl Pts',(-12.4040626064597,13.2248094693827,465.346209595194));
#13722=CARTESIAN_POINT('Ctrl Pts',(-13.1976744186047,12.44352458941,464.546209595194));
#13723=CARTESIAN_POINT('Ctrl Pts',(-12.9946426736236,12.6697216470157,464.546209595194));
#13724=CARTESIAN_POINT('Ctrl Pts',(-12.6877533107556,12.9742099394735,464.640330366534));
#13725=CARTESIAN_POINT('Ctrl Pts',(-12.4087500684403,13.2210165003895,465.020640264799));
#13726=CARTESIAN_POINT('Ctrl Pts',(-12.3604651162791,13.2622157662295,465.237293355737));
#13727=CARTESIAN_POINT('Ctrl Pts',(-12.3604651162791,13.2622157662295,465.346209595194));
#13728=CARTESIAN_POINT('',(-12.5,12.9586405314001,465.346209595194));
#13729=CARTESIAN_POINT('',(-12.9,12.1763356291059,464.946209595194));
#13730=CARTESIAN_POINT('Ctrl Pts',(-12.9,12.1763356291059,464.946209595194));
#13731=CARTESIAN_POINT('Ctrl Pts',(-12.8029959440646,12.3924794841513,464.946209595194));
#13732=CARTESIAN_POINT('Ctrl Pts',(-12.6563710262499,12.683434963611,464.993269980864));
#13733=CARTESIAN_POINT('Ctrl Pts',(-12.5230694771437,12.9192723440419,465.183424929997));
#13734=CARTESIAN_POINT('Ctrl Pts',(-12.5,12.9586405314001,465.291751475466));
#13735=CARTESIAN_POINT('Ctrl Pts',(-12.5,12.9586405314001,465.346209595194));
#13736=CARTESIAN_POINT('',(-12.3604651162791,13.2622157662296,465.346209595194));
#13737=CARTESIAN_POINT('Origin',(-12.1,12.9586405314001,465.346209595194));
#13738=CARTESIAN_POINT('',(-13.1976744186047,12.44352458941,464.546209595194));
#13739=CARTESIAN_POINT('Ctrl Pts',(-12.3604651162791,13.2622157662295,465.346209595194));
#13740=CARTESIAN_POINT('Ctrl Pts',(-12.3604651162791,13.2622157662295,465.237293355737));
#13741=CARTESIAN_POINT('Ctrl Pts',(-12.4087500684403,13.2210165003895,465.020640264799));
#13742=CARTESIAN_POINT('Ctrl Pts',(-12.6877533107556,12.9742099394735,464.640330366534));
#13743=CARTESIAN_POINT('Ctrl Pts',(-12.9946426736236,12.6697216470157,464.546209595194));
#13744=CARTESIAN_POINT('Ctrl Pts',(-13.1976744186047,12.44352458941,464.546209595194));
#13745=CARTESIAN_POINT('Origin',(-12.9,12.1763356291059,464.546209595194));
#13746=CARTESIAN_POINT('Ctrl Pts',(-12.5,-0.0950945662644365,465.346209595194));
#13747=CARTESIAN_POINT('Ctrl Pts',(-12.5,-0.0950945662644367,465.29175196324));
#13748=CARTESIAN_POINT('Ctrl Pts',(-12.5230712817632,-0.055723237524717,
465.183423780398));
#13749=CARTESIAN_POINT('Ctrl Pts',(-12.6563723650316,0.180113321251888,
464.993272151286));
#13750=CARTESIAN_POINT('Ctrl Pts',(-12.8029968129178,0.471068416957768,
464.946209595194));
#13751=CARTESIAN_POINT('Ctrl Pts',(-12.9,0.687210336029828,464.946209595194));
#13752=CARTESIAN_POINT('Ctrl Pts',(-12.5,-0.152539950707804,465.346209595194));
#13753=CARTESIAN_POINT('Ctrl Pts',(-12.5,-0.152539950707804,465.285050846981));
#13754=CARTESIAN_POINT('Ctrl Pts',(-12.5288205011401,-0.113503572746219,
465.163347579182));
#13755=CARTESIAN_POINT('Ctrl Pts',(-12.6938347824102,0.119709443021527,
464.958571481921));
#13756=CARTESIAN_POINT('Ctrl Pts',(-12.8697235920656,0.406597322726993,
464.926883606465));
#13757=CARTESIAN_POINT('Ctrl Pts',(-12.9779309805542,0.617260429795526,
464.946209595194));
#13758=CARTESIAN_POINT('Ctrl Pts',(-12.4748409267651,-0.267385909988173,
465.346209595194));
#13759=CARTESIAN_POINT('Ctrl Pts',(-12.4748409267651,-0.267385909988173,
465.268198488334));
#13760=CARTESIAN_POINT('Ctrl Pts',(-12.5140076158955,-0.229108956409242,
465.113238091813));
#13761=CARTESIAN_POINT('Ctrl Pts',(-12.7386250832635,-0.000953121784120126,
464.854841435699));
#13762=CARTESIAN_POINT('Ctrl Pts',(-12.9815617779372,0.277631354593801,
464.82402503853));
#13763=CARTESIAN_POINT('Ctrl Pts',(-13.1330575681819,0.478020679674991,
464.859380702438));
#13764=CARTESIAN_POINT('Ctrl Pts',(-12.4040626064597,-0.361263504247002,
465.346209595194));
#13765=CARTESIAN_POINT('Ctrl Pts',(-12.4040626064597,-0.361263504247002,
465.247600832946));
#13766=CARTESIAN_POINT('Ctrl Pts',(-12.4497792119805,-0.32152443178383,
465.051464677961));
#13767=CARTESIAN_POINT('Ctrl Pts',(-12.7145981275216,-0.0846988078642869,
464.711884088098));
#13768=CARTESIAN_POINT('Ctrl Pts',(-13.00568558232,0.206714425128216,464.638779800898));
#13769=CARTESIAN_POINT('Ctrl Pts',(-13.1976744186047,0.42002137572574,464.650929350314));
#13770=CARTESIAN_POINT('Ctrl Pts',(-12.3604651162791,-0.398669801093845,
465.346209595194));
#13771=CARTESIAN_POINT('Ctrl Pts',(-12.3604651162791,-0.398669801093846,
465.237294331286));
#13772=CARTESIAN_POINT('Ctrl Pts',(-12.4087538455509,-0.357467247761575,
465.020637965603));
#13773=CARTESIAN_POINT('Ctrl Pts',(-12.6877561128567,-0.110661546716286,
464.640334707378));
#13774=CARTESIAN_POINT('Ctrl Pts',(-12.9946444921535,0.1938263441387,464.546209595194));
#13775=CARTESIAN_POINT('Ctrl Pts',(-13.1976744186047,0.42002137572574,464.546209595194));
#13776=CARTESIAN_POINT('',(-13.1976744186047,0.420021375725734,464.546209595194));
#13777=CARTESIAN_POINT('',(-12.3604651162791,-0.398669801093845,465.346209595194));
#13778=CARTESIAN_POINT('Ctrl Pts',(-13.1976744186047,0.42002137572574,464.546209595194));
#13779=CARTESIAN_POINT('Ctrl Pts',(-12.9946444921535,0.1938263441387,464.546209595194));
#13780=CARTESIAN_POINT('Ctrl Pts',(-12.6877561128567,-0.110661546716286,
464.640334707378));
#13781=CARTESIAN_POINT('Ctrl Pts',(-12.4087538455509,-0.357467247761575,
465.020637965603));
#13782=CARTESIAN_POINT('Ctrl Pts',(-12.3604651162791,-0.398669801093846,
465.237294331286));
#13783=CARTESIAN_POINT('Ctrl Pts',(-12.3604651162791,-0.398669801093845,
465.346209595194));
#13784=CARTESIAN_POINT('',(-12.5,-0.0950945662644354,465.346209595194));
#13785=CARTESIAN_POINT('Origin',(-12.1,-0.0950945662644354,465.346209595194));
#13786=CARTESIAN_POINT('',(-12.9,0.687210336029827,464.946209595194));
#13787=CARTESIAN_POINT('Ctrl Pts',(-12.5,-0.0950945662644365,465.346209595194));
#13788=CARTESIAN_POINT('Ctrl Pts',(-12.5,-0.0950945662644367,465.29175196324));
#13789=CARTESIAN_POINT('Ctrl Pts',(-12.5230712817632,-0.055723237524717,
465.183423780398));
#13790=CARTESIAN_POINT('Ctrl Pts',(-12.6563723650316,0.180113321251888,
464.993272151286));
#13791=CARTESIAN_POINT('Ctrl Pts',(-12.8029968129178,0.471068416957768,
464.946209595194));
#13792=CARTESIAN_POINT('Ctrl Pts',(-12.9,0.687210336029828,464.946209595194));
#13793=CARTESIAN_POINT('Origin',(-12.9,0.687210336029829,464.546209595194));
#13794=CARTESIAN_POINT('Origin',(-12.1,12.9586405314001,462.946209595194));
#13795=CARTESIAN_POINT('',(-12.5,12.9586405314001,476.446209595194));
#13796=CARTESIAN_POINT('',(-12.3604651162791,13.2622157662296,476.446209595194));
#13797=CARTESIAN_POINT('Origin',(-12.1,12.9586405314001,476.446209595194));
#13798=CARTESIAN_POINT('',(-12.3604651162791,13.2622157662296,462.946209595194));
#13799=CARTESIAN_POINT('',(-12.5,12.9586405314001,462.946209595194));
#13800=CARTESIAN_POINT('Ctrl Pts',(-12.5,12.9586405314001,476.446209595194));
#13801=CARTESIAN_POINT('Ctrl Pts',(-12.5,12.9586405314002,476.853861255764));
#13802=CARTESIAN_POINT('Ctrl Pts',(-12.5,12.7121305874131,477.448240925556));
#13803=CARTESIAN_POINT('Ctrl Pts',(-12.5,11.6095151659742,478.389250767395));
#13804=CARTESIAN_POINT('Ctrl Pts',(-12.5,10.5470763037083,478.546209595194));
#13805=CARTESIAN_POINT('Ctrl Pts',(-12.5,9.73177298256796,478.546209595194));
#13806=CARTESIAN_POINT('Ctrl Pts',(-12.5,13.0160859158435,476.446209595194));
#13807=CARTESIAN_POINT('Ctrl Pts',(-12.5,13.0160859158436,476.868556690467));
#13808=CARTESIAN_POINT('Ctrl Pts',(-12.499798919425,12.7644563196739,477.484521897399));
#13809=CARTESIAN_POINT('Ctrl Pts',(-12.4999487018801,11.6399911364717,478.465534436156));
#13810=CARTESIAN_POINT('Ctrl Pts',(-12.4996309047003,10.5575748644185,478.639497203128));
#13811=CARTESIAN_POINT('Ctrl Pts',(-12.5,9.73177298256796,478.650929350314));
#13812=CARTESIAN_POINT('Ctrl Pts',(-12.4748408382406,13.1309318344346,476.446209595194));
#13813=CARTESIAN_POINT('Ctrl Pts',(-12.4748408382406,13.1309318344347,476.897925676163));
#13814=CARTESIAN_POINT('Ctrl Pts',(-12.4714917573037,12.8690363604298,477.557273431096));
#13815=CARTESIAN_POINT('Ctrl Pts',(-12.4543886115941,11.7008031686518,478.618026795867));
#13816=CARTESIAN_POINT('Ctrl Pts',(-12.4330371840754,10.5783878700328,478.826112000052));
#13817=CARTESIAN_POINT('Ctrl Pts',(-12.4131704002205,9.73177298256796,478.859379995414));
#13818=CARTESIAN_POINT('Ctrl Pts',(-12.4040626064597,13.2248094693827,476.446209595194));
#13819=CARTESIAN_POINT('Ctrl Pts',(-12.4040626064597,13.2248094693828,476.921954463457));
#13820=CARTESIAN_POINT('Ctrl Pts',(-12.3915856347517,12.9517896616252,477.615790277435));
#13821=CARTESIAN_POINT('Ctrl Pts',(-12.3316250640951,11.7391724081509,478.725157762151));
#13822=CARTESIAN_POINT('Ctrl Pts',(-12.2613563482675,10.587188239976,478.928024760507));
#13823=CARTESIAN_POINT('Ctrl Pts',(-12.2047197551197,9.73177298256796,478.946209595194));
#13824=CARTESIAN_POINT('Ctrl Pts',(-12.3604651162791,13.2622157662295,476.446209595194));
#13825=CARTESIAN_POINT('Ctrl Pts',(-12.3604651162791,13.2622157662296,476.931509191111));
#13826=CARTESIAN_POINT('Ctrl Pts',(-12.342893213559,12.9832980857263,477.639104036101));
#13827=CARTESIAN_POINT('Ctrl Pts',(-12.2600218813812,11.7488052197396,478.759353847815));
#13828=CARTESIAN_POINT('Ctrl Pts',(-12.167925862495,10.5871040441072,478.946209595194));
#13829=CARTESIAN_POINT('Ctrl Pts',(-12.1,9.73177298256796,478.946209595194));
#13830=CARTESIAN_POINT('',(-12.5,9.73177298256795,478.546209595194));
#13831=CARTESIAN_POINT('',(-12.1,9.73177298256795,478.946209595194));
#13832=CARTESIAN_POINT('Origin',(-12.1,9.73177298256795,478.546209595194));
#13833=CARTESIAN_POINT('Ctrl Pts',(-12.1,9.73177298256796,478.946209595194));
#13834=CARTESIAN_POINT('Ctrl Pts',(-12.167925862495,10.5871040441072,478.946209595194));
#13835=CARTESIAN_POINT('Ctrl Pts',(-12.2600218813812,11.7488052197396,478.759353847815));
#13836=CARTESIAN_POINT('Ctrl Pts',(-12.342893213559,12.9832980857263,477.639104036101));
#13837=CARTESIAN_POINT('Ctrl Pts',(-12.3604651162791,13.2622157662296,476.931509191111));
#13838=CARTESIAN_POINT('Ctrl Pts',(-12.3604651162791,13.2622157662295,476.446209595194));
#13839=CARTESIAN_POINT('Ctrl Pts',(-12.5,12.9586405314001,476.446209595194));
#13840=CARTESIAN_POINT('Ctrl Pts',(-12.5,12.9586405314002,476.853861255764));
#13841=CARTESIAN_POINT('Ctrl Pts',(-12.5,12.7121305874131,477.448240925556));
#13842=CARTESIAN_POINT('Ctrl Pts',(-12.5,11.6095151659742,478.389250767395));
#13843=CARTESIAN_POINT('Ctrl Pts',(-12.5,10.5470763037083,478.546209595194));
#13844=CARTESIAN_POINT('Ctrl Pts',(-12.5,9.73177298256796,478.546209595194));
#13845=CARTESIAN_POINT('Origin',(-12.1,9.78587494881754,478.546209595194));
#13846=CARTESIAN_POINT('',(-12.5,3.13177298256785,478.546209595194));
#13847=CARTESIAN_POINT('',(-12.1,3.13177298256785,478.946209595194));
#13848=CARTESIAN_POINT('Origin',(-12.1,3.13177298256785,478.546209595194));
#13849=CARTESIAN_POINT('',(-12.1,9.78587494881754,478.946209595194));
#13850=CARTESIAN_POINT('',(-12.5,9.78587494881754,478.546209595194));
#13851=CARTESIAN_POINT('Ctrl Pts',(-12.5,3.13177298256785,478.546209595194));
#13852=CARTESIAN_POINT('Ctrl Pts',(-12.5,2.52026774111634,478.546209595194));
#13853=CARTESIAN_POINT('Ctrl Pts',(-12.5,1.48936227736903,478.433754771008));
#13854=CARTESIAN_POINT('Ctrl Pts',(-12.5,0.244282023002687,477.649528864133));
#13855=CARTESIAN_POINT('Ctrl Pts',(-12.5,-0.0950945662644376,476.853879756162));
#13856=CARTESIAN_POINT('Ctrl Pts',(-12.5,-0.0950945662644376,476.446209595194));
#13857=CARTESIAN_POINT('Ctrl Pts',(-12.5,3.13177298256785,478.650929350314));
#13858=CARTESIAN_POINT('Ctrl Pts',(-12.4997231659623,2.51239346324273,478.642354850807));
#13859=CARTESIAN_POINT('Ctrl Pts',(-12.4998708957056,1.46352149007596,478.513649678176));
#13860=CARTESIAN_POINT('Ctrl Pts',(-12.4997435365771,0.193842442444793,
477.69306379392));
#13861=CARTESIAN_POINT('Ctrl Pts',(-12.5,-0.152539950707804,476.868575857786));
#13862=CARTESIAN_POINT('Ctrl Pts',(-12.5,-0.152539950707804,476.446209595194));
#13863=CARTESIAN_POINT('Ctrl Pts',(-12.4131706406899,3.13177298256785,478.859380235884));
#13864=CARTESIAN_POINT('Ctrl Pts',(-12.4280714047896,2.49678300061667,478.834428107014));
#13865=CARTESIAN_POINT('Ctrl Pts',(-12.4502945445776,1.41200273935032,478.673426816548));
#13866=CARTESIAN_POINT('Ctrl Pts',(-12.4703420994035,0.0930418380396119,
477.780378953069));
#13867=CARTESIAN_POINT('Ctrl Pts',(-12.4748408683491,-0.267385883137938,
476.89794617633));
#13868=CARTESIAN_POINT('Ctrl Pts',(-12.4748408683491,-0.267385883137938,
476.446209595194));
#13869=CARTESIAN_POINT('Ctrl Pts',(-12.2047197551197,3.13177298256785,478.946209595194));
#13870=CARTESIAN_POINT('Ctrl Pts',(-12.2471991277284,2.49018242361983,478.932570350219));
#13871=CARTESIAN_POINT('Ctrl Pts',(-12.3174618184511,1.38194921130776,478.780697709241));
#13872=CARTESIAN_POINT('Ctrl Pts',(-12.387272273891,0.014706061216163,477.850660975865));
#13873=CARTESIAN_POINT('Ctrl Pts',(-12.4040626064597,-0.361263504247001,
476.921976054119));
#13874=CARTESIAN_POINT('Ctrl Pts',(-12.4040626064597,-0.361263504247001,
476.446209595194));
#13875=CARTESIAN_POINT('Ctrl Pts',(-12.1,3.13177298256785,478.946209595194));
#13876=CARTESIAN_POINT('Ctrl Pts',(-12.1509467088736,2.49024557338726,478.946209595194));
#13877=CARTESIAN_POINT('Ctrl Pts',(-12.2408287043769,1.37587602390371,478.812334804496));
#13878=CARTESIAN_POINT('Ctrl Pts',(-12.3367447800671,-0.0143093659240391,
477.878732534407));
#13879=CARTESIAN_POINT('Ctrl Pts',(-12.3604651162791,-0.398669801093845,
476.931531215393));
#13880=CARTESIAN_POINT('Ctrl Pts',(-12.3604651162791,-0.398669801093845,
476.446209595194));
#13881=CARTESIAN_POINT('',(-12.5,-0.0950945662644376,476.446209595194));
#13882=CARTESIAN_POINT('',(-12.3604651162791,-0.398669801093845,476.446209595194));
#13883=CARTESIAN_POINT('Origin',(-12.1,-0.0950945662644365,476.446209595194));
#13884=CARTESIAN_POINT('Ctrl Pts',(-12.3604651162791,-0.398669801093845,
476.446209595194));
#13885=CARTESIAN_POINT('Ctrl Pts',(-12.3604651162791,-0.398669801093845,
476.931531215393));
#13886=CARTESIAN_POINT('Ctrl Pts',(-12.3367447800671,-0.0143093659240391,
477.878732534407));
#13887=CARTESIAN_POINT('Ctrl Pts',(-12.2408287043769,1.37587602390371,478.812334804496));
#13888=CARTESIAN_POINT('Ctrl Pts',(-12.1509467088736,2.49024557338726,478.946209595194));
#13889=CARTESIAN_POINT('Ctrl Pts',(-12.1,3.13177298256785,478.946209595194));
#13890=CARTESIAN_POINT('Ctrl Pts',(-12.5,3.13177298256785,478.546209595194));
#13891=CARTESIAN_POINT('Ctrl Pts',(-12.5,2.52026774111634,478.546209595194));
#13892=CARTESIAN_POINT('Ctrl Pts',(-12.5,1.48936227736903,478.433754771008));
#13893=CARTESIAN_POINT('Ctrl Pts',(-12.5,0.244282023002687,477.649528864133));
#13894=CARTESIAN_POINT('Ctrl Pts',(-12.5,-0.0950945662644376,476.853879756162));
#13895=CARTESIAN_POINT('Ctrl Pts',(-12.5,-0.0950945662644376,476.446209595194));
#13896=CARTESIAN_POINT('Origin',(-12.1,-0.0950945662644354,462.946209595194));
#13897=CARTESIAN_POINT('',(-12.3604651162791,-0.398669801093845,462.946209595194));
#13898=CARTESIAN_POINT('',(-12.5,-0.0950945662644354,462.946209595194));
#13899=CARTESIAN_POINT('Origin',(-12.9,9.78587494881754,465.346209595194));
#13900=CARTESIAN_POINT('',(-12.5,9.78587494881754,465.346209595194));
#13901=CARTESIAN_POINT('',(-12.9,9.78587494881754,464.946209595194));
#13902=CARTESIAN_POINT('Origin',(-6.5,6.43177298256785,464.546209595194));
#13903=CARTESIAN_POINT('',(-15.5,6.43177298256785,464.546209595194));
#13904=CARTESIAN_POINT('Origin',(-6.5,6.43177298256785,464.546209595194));
#13905=CARTESIAN_POINT('Origin',(-6.5,6.43177298256785,464.546209595194));
#13906=CARTESIAN_POINT('Origin',(-6.5,6.43177298256785,464.946209595194));
#13907=CARTESIAN_POINT('Origin',(-6.5,6.43177298256785,478.946209595194));
#13908=CARTESIAN_POINT('',(-0.900000000000017,3.13177298256776,478.946209595194));
#13909=CARTESIAN_POINT('Origin',(-6.5,6.43177298256785,478.946209595194));
#13910=CARTESIAN_POINT('',(-0.899999999999997,9.73177298256785,478.946209595194));
#13911=CARTESIAN_POINT('',(-0.899999999999997,3.07767101631817,478.946209595194));
#13912=CARTESIAN_POINT('Origin',(-6.5,6.43177298256785,478.946209595194));
#13913=CARTESIAN_POINT('Origin',(-6.5,6.43177298256785,476.446209595194));
#13914=CARTESIAN_POINT('',(-0.639534883720928,-0.398669801093843,476.446209595194));
#13915=CARTESIAN_POINT('Origin',(-6.5,6.43177298256785,476.446209595194));
#13916=CARTESIAN_POINT('Ctrl Pts',(-0.899999999999989,3.13177298256775,
478.946209595194));
#13917=CARTESIAN_POINT('Ctrl Pts',(-0.83207413779171,2.27644192463902,478.946209595194));
#13918=CARTESIAN_POINT('Ctrl Pts',(-0.739978110974983,1.11474130806174,
478.759354402431));
#13919=CARTESIAN_POINT('Ctrl Pts',(-0.657106776481008,-0.119751885582937,
477.639104541356));
#13920=CARTESIAN_POINT('Ctrl Pts',(-0.639534883720916,-0.398669801093799,
476.93150918906));
#13921=CARTESIAN_POINT('Ctrl Pts',(-0.639534883720934,-0.398669801093842,
476.446209595194));
#13922=CARTESIAN_POINT('Origin',(-12.5,13.1399769150672,478.946209595194));
#13923=CARTESIAN_POINT('',(-12.5,10.4317729825678,471.090577685893));
#13924=CARTESIAN_POINT('Origin',(-12.5,6.43177298256785,471.090577685893));
#13925=CARTESIAN_POINT('Origin',(-14.,6.43177298256785,464.946209595194));
#13926=CARTESIAN_POINT('Ctrl Pts',(-0.499999999999996,12.9586405314001,
465.346209595194));
#13927=CARTESIAN_POINT('Ctrl Pts',(-0.499999999999997,12.9586405314001,
465.291751963028));
#13928=CARTESIAN_POINT('Ctrl Pts',(-0.476928716540935,12.9192691993652,
465.183423779369));
#13929=CARTESIAN_POINT('Ctrl Pts',(-0.34362763610145,12.6834326448933,464.993272154916));
#13930=CARTESIAN_POINT('Ctrl Pts',(-0.197003187459576,12.3924775490188,
464.946209595194));
#13931=CARTESIAN_POINT('Ctrl Pts',(-0.0999999999999975,12.1763356291059,
464.946209595194));
#13932=CARTESIAN_POINT('Ctrl Pts',(-0.499999999999996,13.0160859158435,
465.346209595194));
#13933=CARTESIAN_POINT('Ctrl Pts',(-0.499999999999997,13.0160859158435,
465.285050846744));
#13934=CARTESIAN_POINT('Ctrl Pts',(-0.471179496785347,12.9770495346129,
465.16334757817));
#13935=CARTESIAN_POINT('Ctrl Pts',(-0.306165219154938,12.7438365231285,
464.958571486081));
#13936=CARTESIAN_POINT('Ctrl Pts',(-0.130276408355345,12.4569486432282,
464.92688360639));
#13937=CARTESIAN_POINT('Ctrl Pts',(-0.0220690194458337,12.2462855353402,
464.946209595194));
#13938=CARTESIAN_POINT('Ctrl Pts',(-0.525159075955398,13.1309318738734,
465.346209595194));
#13939=CARTESIAN_POINT('Ctrl Pts',(-0.525159075955398,13.1309318738734,
465.26819848803));
#13940=CARTESIAN_POINT('Ctrl Pts',(-0.4859923865512,13.0926549146057,465.113238086588));
#13941=CARTESIAN_POINT('Ctrl Pts',(-0.261374923085867,12.8644990852749,
464.85484143889));
#13942=CARTESIAN_POINT('Ctrl Pts',(-0.0184382388215931,12.585914596808,
464.824025016665));
#13943=CARTESIAN_POINT('Ctrl Pts',(0.133057552012535,12.3855252709472,464.859380680711));
#13944=CARTESIAN_POINT('Ctrl Pts',(-0.595937393540275,13.2248094693827,
465.346209595194));
#13945=CARTESIAN_POINT('Ctrl Pts',(-0.595937393540275,13.2248094693827,
465.247600832562));
#13946=CARTESIAN_POINT('Ctrl Pts',(-0.550220784700754,13.1850703935657,
465.051464676199));
#13947=CARTESIAN_POINT('Ctrl Pts',(-0.285401874822712,12.9482447739809,
464.711884094779));
#13948=CARTESIAN_POINT('Ctrl Pts',(0.00568558157314103,12.6568315408373,
464.63877980085));
#13949=CARTESIAN_POINT('Ctrl Pts',(0.197674418604646,12.44352458941,464.650929350314));
#13950=CARTESIAN_POINT('Ctrl Pts',(-0.639534883720927,13.2622157662295,
465.346209595194));
#13951=CARTESIAN_POINT('Ctrl Pts',(-0.639534883720927,13.2622157662295,
465.237294330863));
#13952=CARTESIAN_POINT('Ctrl Pts',(-0.591246150899638,13.2210132094488,
465.020637963544));
#13953=CARTESIAN_POINT('Ctrl Pts',(-0.31224388951466,12.9742075129084,464.640334714638));
#13954=CARTESIAN_POINT('Ctrl Pts',(-0.00535550863633265,12.6697196218769,
464.546209595194));
#13955=CARTESIAN_POINT('Ctrl Pts',(0.197674418604645,12.44352458941,464.546209595194));
#13956=CARTESIAN_POINT('',(0.197674418604654,12.44352458941,464.546209595194));
#13957=CARTESIAN_POINT('',(-0.639534883720926,13.2622157662295,465.346209595194));
#13958=CARTESIAN_POINT('Ctrl Pts',(0.197674418604645,12.44352458941,464.546209595194));
#13959=CARTESIAN_POINT('Ctrl Pts',(-0.00535550863633265,12.6697196218769,
464.546209595194));
#13960=CARTESIAN_POINT('Ctrl Pts',(-0.31224388951466,12.9742075129084,464.640334714638));
#13961=CARTESIAN_POINT('Ctrl Pts',(-0.591246150899638,13.2210132094488,
465.020637963544));
#13962=CARTESIAN_POINT('Ctrl Pts',(-0.639534883720927,13.2622157662295,
465.237294330863));
#13963=CARTESIAN_POINT('Ctrl Pts',(-0.639534883720927,13.2622157662295,
465.346209595194));
#13964=CARTESIAN_POINT('',(-0.499999999999997,12.9586405314001,465.346209595194));
#13965=CARTESIAN_POINT('Origin',(-0.899999999999996,12.9586405314001,465.346209595194));
#13966=CARTESIAN_POINT('',(-0.0999999999999979,12.1763356291059,464.946209595194));
#13967=CARTESIAN_POINT('Ctrl Pts',(-0.499999999999996,12.9586405314001,
465.346209595194));
#13968=CARTESIAN_POINT('Ctrl Pts',(-0.499999999999997,12.9586405314001,
465.291751963028));
#13969=CARTESIAN_POINT('Ctrl Pts',(-0.476928716540935,12.9192691993652,
465.183423779369));
#13970=CARTESIAN_POINT('Ctrl Pts',(-0.34362763610145,12.6834326448933,464.993272154916));
#13971=CARTESIAN_POINT('Ctrl Pts',(-0.197003187459576,12.3924775490188,
464.946209595194));
#13972=CARTESIAN_POINT('Ctrl Pts',(-0.0999999999999975,12.1763356291059,
464.946209595194));
#13973=CARTESIAN_POINT('Origin',(-0.0999999999999979,12.1763356291059,464.546209595194));
#13974=CARTESIAN_POINT('Ctrl Pts',(-0.0999999999999936,0.687210336029823,
464.946209595194));
#13975=CARTESIAN_POINT('Ctrl Pts',(-0.197004053805406,0.471066485730349,
464.946209595194));
#13976=CARTESIAN_POINT('Ctrl Pts',(-0.343628961915439,0.180111016895773,
464.993269988545));
#13977=CARTESIAN_POINT('Ctrl Pts',(-0.476930512726993,-0.0557263627151083,
465.183424919342));
#13978=CARTESIAN_POINT('Ctrl Pts',(-0.499999999999998,-0.0950945662644381,
465.291751476661));
#13979=CARTESIAN_POINT('Ctrl Pts',(-0.499999999999998,-0.0950945662644381,
465.346209595194));
#13980=CARTESIAN_POINT('Ctrl Pts',(-0.0220690194458293,0.617260429795521,
464.946209595194));
#13981=CARTESIAN_POINT('Ctrl Pts',(-0.130277374767095,0.406595440452743,
464.926883433788));
#13982=CARTESIAN_POINT('Ctrl Pts',(-0.306166894624085,0.119707152456133,
464.95856892495));
#13983=CARTESIAN_POINT('Ctrl Pts',(-0.471181729397159,-0.113506665586292,
465.16334876686));
#13984=CARTESIAN_POINT('Ctrl Pts',(-0.499999999999998,-0.152539950707803,
465.285050300528));
#13985=CARTESIAN_POINT('Ctrl Pts',(-0.499999999999998,-0.152539950707804,
465.346209595194));
#13986=CARTESIAN_POINT('Ctrl Pts',(0.133057850423733,0.47802042633817,464.859381081701));
#13987=CARTESIAN_POINT('Ctrl Pts',(-0.0184392934354909,0.277629310778949,
464.82402510189));
#13988=CARTESIAN_POINT('Ctrl Pts',(-0.261377121062116,-0.000955430391377806,
464.854838190806));
#13989=CARTESIAN_POINT('Ctrl Pts',(-0.485995323452632,-0.229112051155817,
465.113239647082));
#13990=CARTESIAN_POINT('Ctrl Pts',(-0.525159025748574,-0.267385931814736,
465.268197791304));
#13991=CARTESIAN_POINT('Ctrl Pts',(-0.525159025748574,-0.267385931814736,
465.346209595194));
#13992=CARTESIAN_POINT('Ctrl Pts',(0.197674418604656,0.420021375725734,
464.650929350314));
#13993=CARTESIAN_POINT('Ctrl Pts',(0.00568386690033115,0.206712519231232,
464.638779692341));
#13994=CARTESIAN_POINT('Ctrl Pts',(-0.28540451322635,-0.0847011369192216,
464.711880110167));
#13995=CARTESIAN_POINT('Ctrl Pts',(-0.550224351095307,-0.32152757410988,
465.051466690852));
#13996=CARTESIAN_POINT('Ctrl Pts',(-0.595937393540273,-0.361263504246996,
465.247599951876));
#13997=CARTESIAN_POINT('Ctrl Pts',(-0.595937393540273,-0.361263504246996,
465.346209595194));
#13998=CARTESIAN_POINT('Ctrl Pts',(0.197674418604656,0.420021375725734,
464.546209595194));
#13999=CARTESIAN_POINT('Ctrl Pts',(-0.0053573219182965,0.193824323086751,
464.546209595194));
#14000=CARTESIAN_POINT('Ctrl Pts',(-0.31224666447418,-0.110663958251744,
464.640330381896));
#14001=CARTESIAN_POINT('Ctrl Pts',(-0.591249910358824,-0.357470518309637,
465.020640243491));
#14002=CARTESIAN_POINT('Ctrl Pts',(-0.639534883720924,-0.398669801093839,
465.237293358129));
#14003=CARTESIAN_POINT('Ctrl Pts',(-0.639534883720924,-0.398669801093839,
465.346209595194));
#14004=CARTESIAN_POINT('',(-0.499999999999998,-0.0950945662644331,465.346209595194));
#14005=CARTESIAN_POINT('',(-0.0999999999999979,0.687210336029828,464.946209595194));
#14006=CARTESIAN_POINT('Ctrl Pts',(-0.0999999999999936,0.687210336029823,
464.946209595194));
#14007=CARTESIAN_POINT('Ctrl Pts',(-0.197004053805406,0.471066485730349,
464.946209595194));
#14008=CARTESIAN_POINT('Ctrl Pts',(-0.343628961915439,0.180111016895773,
464.993269988545));
#14009=CARTESIAN_POINT('Ctrl Pts',(-0.476930512726993,-0.0557263627151083,
465.183424919342));
#14010=CARTESIAN_POINT('Ctrl Pts',(-0.499999999999998,-0.0950945662644381,
465.291751476661));
#14011=CARTESIAN_POINT('Ctrl Pts',(-0.499999999999998,-0.0950945662644381,
465.346209595194));
#14012=CARTESIAN_POINT('',(-0.639534883720928,-0.398669801093843,465.346209595194));
#14013=CARTESIAN_POINT('Origin',(-0.899999999999999,-0.0950945662644331,
465.346209595194));
#14014=CARTESIAN_POINT('',(0.197674418604655,0.420021375725734,464.546209595194));
#14015=CARTESIAN_POINT('Ctrl Pts',(-0.639534883720924,-0.398669801093839,
465.346209595194));
#14016=CARTESIAN_POINT('Ctrl Pts',(-0.639534883720924,-0.398669801093839,
465.237293358129));
#14017=CARTESIAN_POINT('Ctrl Pts',(-0.591249910358824,-0.357470518309637,
465.020640243491));
#14018=CARTESIAN_POINT('Ctrl Pts',(-0.31224666447418,-0.110663958251744,
464.640330381896));
#14019=CARTESIAN_POINT('Ctrl Pts',(-0.0053573219182965,0.193824323086751,
464.546209595194));
#14020=CARTESIAN_POINT('Ctrl Pts',(0.197674418604656,0.420021375725734,
464.546209595194));
#14021=CARTESIAN_POINT('Origin',(-0.0999999999999979,0.687210336029827,
464.546209595194));
#14022=CARTESIAN_POINT('Origin',(-0.899999999999999,-0.0950945662644331,
462.946209595194));
#14023=CARTESIAN_POINT('',(-0.499999999999998,-0.0950945662644331,476.446209595194));
#14024=CARTESIAN_POINT('Origin',(-0.899999999999999,-0.0950945662644331,
476.446209595194));
#14025=CARTESIAN_POINT('',(-0.639534883720928,-0.398669801093843,462.946209595194));
#14026=CARTESIAN_POINT('',(-0.499999999999998,-0.0950945662644331,462.946209595194));
#14027=CARTESIAN_POINT('Ctrl Pts',(-0.499999999999998,-0.0950945662644388,
476.446209595194));
#14028=CARTESIAN_POINT('Ctrl Pts',(-0.499999999999998,-0.0950945662643835,
476.853861254042));
#14029=CARTESIAN_POINT('Ctrl Pts',(-0.499999999999998,0.151415578718571,
477.44824134997));
#14030=CARTESIAN_POINT('Ctrl Pts',(-0.499999999999998,1.25403127909223,
478.389251233274));
#14031=CARTESIAN_POINT('Ctrl Pts',(-0.499999999999998,2.31646966486893,
478.546209595194));
#14032=CARTESIAN_POINT('Ctrl Pts',(-0.499999999999998,3.13177298256775,
478.546209595194));
#14033=CARTESIAN_POINT('Ctrl Pts',(-0.5,-0.152539950707805,476.446209595194));
#14034=CARTESIAN_POINT('Ctrl Pts',(-0.499999999999997,-0.152539950707749,
476.868556688683));
#14035=CARTESIAN_POINT('Ctrl Pts',(-0.500201055627566,0.0990898464205717,
477.484522337147));
#14036=CARTESIAN_POINT('Ctrl Pts',(-0.5000512665282,1.22355531214914,478.465534919309));
#14037=CARTESIAN_POINT('Ctrl Pts',(-0.50036909529811,2.30597110420312,478.639497203177));
#14038=CARTESIAN_POINT('Ctrl Pts',(-0.499999999999998,3.13177298256775,
478.650929350314));
#14039=CARTESIAN_POINT('Ctrl Pts',(-0.52515909003033,-0.267385902268368,
476.446209595194));
#14040=CARTESIAN_POINT('Ctrl Pts',(-0.525159090030321,-0.267385902268311,
476.897925674254));
#14041=CARTESIAN_POINT('Ctrl Pts',(-0.528508029696729,-0.00549022311513094,
477.557274036841));
#14042=CARTESIAN_POINT('Ctrl Pts',(-0.545611187563797,1.16274325449317,
478.618027424828));
#14043=CARTESIAN_POINT('Ctrl Pts',(-0.566962243125236,2.28515809867657,
478.826112573076));
#14044=CARTESIAN_POINT('Ctrl Pts',(-0.586829026896253,3.13177298256775,
478.859380568298));
#14045=CARTESIAN_POINT('Ctrl Pts',(-0.595937393540281,-0.361263504246999,
476.446209595194));
#14046=CARTESIAN_POINT('Ctrl Pts',(-0.595937393540267,-0.361263504246951,
476.921954461446));
#14047=CARTESIAN_POINT('Ctrl Pts',(-0.608414354070092,-0.0882434735480379,
477.615790786554));
#14048=CARTESIAN_POINT('Ctrl Pts',(-0.668374925052943,1.12437409329788,
478.725158324453));
#14049=CARTESIAN_POINT('Ctrl Pts',(-0.738643651971611,2.27635772877052,
478.928024760584));
#14050=CARTESIAN_POINT('Ctrl Pts',(-0.795280244880331,3.13177298256775,
478.946209595194));
#14051=CARTESIAN_POINT('Ctrl Pts',(-0.639534883720934,-0.398669801093842,
476.446209595194));
#14052=CARTESIAN_POINT('Ctrl Pts',(-0.639534883720916,-0.398669801093799,
476.93150918906));
#14053=CARTESIAN_POINT('Ctrl Pts',(-0.657106776481008,-0.119751885582937,
477.639104541356));
#14054=CARTESIAN_POINT('Ctrl Pts',(-0.739978110974983,1.11474130806174,
478.759354402431));
#14055=CARTESIAN_POINT('Ctrl Pts',(-0.83207413779171,2.27644192463902,478.946209595194));
#14056=CARTESIAN_POINT('Ctrl Pts',(-0.899999999999989,3.13177298256775,
478.946209595194));
#14057=CARTESIAN_POINT('',(-0.499999999999998,3.13177298256775,478.546209595194));
#14058=CARTESIAN_POINT('Origin',(-0.899999999999999,3.13177298256775,478.546209595194));
#14059=CARTESIAN_POINT('Ctrl Pts',(-0.499999999999998,-0.0950945662644388,
476.446209595194));
#14060=CARTESIAN_POINT('Ctrl Pts',(-0.499999999999998,-0.0950945662643835,
476.853861254042));
#14061=CARTESIAN_POINT('Ctrl Pts',(-0.499999999999998,0.151415578718571,
477.44824134997));
#14062=CARTESIAN_POINT('Ctrl Pts',(-0.499999999999998,1.25403127909223,
478.389251233274));
#14063=CARTESIAN_POINT('Ctrl Pts',(-0.499999999999998,2.31646966486893,
478.546209595194));
#14064=CARTESIAN_POINT('Ctrl Pts',(-0.499999999999998,3.13177298256775,
478.546209595194));
#14065=CARTESIAN_POINT('Origin',(-0.899999999999997,3.07767101631817,478.546209595194));
#14066=CARTESIAN_POINT('',(-0.499999999999997,9.73177298256785,478.546209595194));
#14067=CARTESIAN_POINT('Origin',(-0.899999999999996,9.73177298256785,478.546209595194));
#14068=CARTESIAN_POINT('',(-0.499999999999998,3.07767101631817,478.546209595194));
#14069=CARTESIAN_POINT('Ctrl Pts',(-0.499999999999997,9.73177298256785,
478.546209595194));
#14070=CARTESIAN_POINT('Ctrl Pts',(-0.499999999999997,10.3432782240194,
478.546209595194));
#14071=CARTESIAN_POINT('Ctrl Pts',(-0.499999999999996,11.3741837099334,
478.433754801363));
#14072=CARTESIAN_POINT('Ctrl Pts',(-0.499999999999996,12.6192639795379,
477.649528900673));
#14073=CARTESIAN_POINT('Ctrl Pts',(-0.499999999999996,12.9586405314001,
476.853879756162));
#14074=CARTESIAN_POINT('Ctrl Pts',(-0.499999999999996,12.9586405314001,
476.446209595194));
#14075=CARTESIAN_POINT('Ctrl Pts',(-0.499999999999997,9.73177298256785,
478.650929350314));
#14076=CARTESIAN_POINT('Ctrl Pts',(-0.500276834037699,10.351152501893,478.642354850807));
#14077=CARTESIAN_POINT('Ctrl Pts',(-0.500129097594821,11.4000244981144,
478.513649710999));
#14078=CARTESIAN_POINT('Ctrl Pts',(-0.500256459014652,12.6697035611434,
477.693063832442));
#14079=CARTESIAN_POINT('Ctrl Pts',(-0.499999999999996,13.0160859158435,
476.868575857786));
#14080=CARTESIAN_POINT('Ctrl Pts',(-0.499999999999996,13.0160859158435,
476.446209595194));
#14081=CARTESIAN_POINT('Ctrl Pts',(-0.586829270574883,9.73177298256785,
478.859380324619));
#14082=CARTESIAN_POINT('Ctrl Pts',(-0.571928506475149,10.366762964519,478.83442819575));
#14083=CARTESIAN_POINT('Ctrl Pts',(-0.549705413042954,11.4515432553218,
478.673426882505));
#14084=CARTESIAN_POINT('Ctrl Pts',(-0.52965786150684,12.7705041717072,477.780379022974));
#14085=CARTESIAN_POINT('Ctrl Pts',(-0.525159120540634,13.1309318533804,
476.89794617633));
#14086=CARTESIAN_POINT('Ctrl Pts',(-0.525159120540634,13.1309318533804,
476.446209595194));
#14087=CARTESIAN_POINT('Ctrl Pts',(-0.795280244880335,9.73177298256785,
478.946209595194));
#14088=CARTESIAN_POINT('Ctrl Pts',(-0.752800872271635,10.3733635415159,
478.932570350219));
#14089=CARTESIAN_POINT('Ctrl Pts',(-0.682538179064161,11.4815967780087,
478.780697751043));
#14090=CARTESIAN_POINT('Ctrl Pts',(-0.612727723661889,12.8488399457344,
477.850661022245));
#14091=CARTESIAN_POINT('Ctrl Pts',(-0.595937393540274,13.2248094693827,
476.921976054119));
#14092=CARTESIAN_POINT('Ctrl Pts',(-0.595937393540274,13.2248094693827,
476.446209595194));
#14093=CARTESIAN_POINT('Ctrl Pts',(-0.899999999999995,9.73177298256785,
478.946209595194));
#14094=CARTESIAN_POINT('Ctrl Pts',(-0.849053291126402,10.3733003917485,
478.946209595194));
#14095=CARTESIAN_POINT('Ctrl Pts',(-0.759171292493971,11.4876699669056,
478.812334840633));
#14096=CARTESIAN_POINT('Ctrl Pts',(-0.663255216974702,12.8778553746618,
477.878732577907));
#14097=CARTESIAN_POINT('Ctrl Pts',(-0.639534883720926,13.2622157662295,
476.931531215393));
#14098=CARTESIAN_POINT('Ctrl Pts',(-0.639534883720926,13.2622157662295,
476.446209595194));
#14099=CARTESIAN_POINT('',(-0.499999999999996,12.9586405314001,476.446209595194));
#14100=CARTESIAN_POINT('',(-0.639534883720926,13.2622157662295,476.446209595194));
#14101=CARTESIAN_POINT('Origin',(-0.899999999999996,12.9586405314001,476.446209595194));
#14102=CARTESIAN_POINT('Ctrl Pts',(-0.639534883720926,13.2622157662295,
476.446209595194));
#14103=CARTESIAN_POINT('Ctrl Pts',(-0.639534883720926,13.2622157662295,
476.931531215393));
#14104=CARTESIAN_POINT('Ctrl Pts',(-0.663255216974702,12.8778553746618,
477.878732577907));
#14105=CARTESIAN_POINT('Ctrl Pts',(-0.759171292493971,11.4876699669056,
478.812334840633));
#14106=CARTESIAN_POINT('Ctrl Pts',(-0.849053291126402,10.3733003917485,
478.946209595194));
#14107=CARTESIAN_POINT('Ctrl Pts',(-0.899999999999995,9.73177298256785,
478.946209595194));
#14108=CARTESIAN_POINT('Ctrl Pts',(-0.499999999999997,9.73177298256785,
478.546209595194));
#14109=CARTESIAN_POINT('Ctrl Pts',(-0.499999999999997,10.3432782240194,
478.546209595194));
#14110=CARTESIAN_POINT('Ctrl Pts',(-0.499999999999996,11.3741837099334,
478.433754801363));
#14111=CARTESIAN_POINT('Ctrl Pts',(-0.499999999999996,12.6192639795379,
477.649528900673));
#14112=CARTESIAN_POINT('Ctrl Pts',(-0.499999999999996,12.9586405314001,
476.853879756162));
#14113=CARTESIAN_POINT('Ctrl Pts',(-0.499999999999996,12.9586405314001,
476.446209595194));
#14114=CARTESIAN_POINT('Origin',(-0.899999999999996,12.9586405314001,462.946209595194));
#14115=CARTESIAN_POINT('',(-0.639534883720926,13.2622157662295,462.946209595194));
#14116=CARTESIAN_POINT('',(-0.499999999999996,12.9586405314001,462.946209595194));
#14117=CARTESIAN_POINT('Origin',(-6.5,6.43177298256785,464.546209595194));
#14118=CARTESIAN_POINT('Origin',(-6.5,6.43177298256785,464.546209595194));
#14119=CARTESIAN_POINT('Origin',(-6.5,6.43177298256785,464.946209595194));
#14120=CARTESIAN_POINT('Origin',(-0.0999999999999979,3.07767101631817,465.346209595194));
#14121=CARTESIAN_POINT('',(-0.499999999999998,3.07767101631817,465.346209595194));
#14122=CARTESIAN_POINT('',(-0.0999999999999979,3.07767101631817,464.946209595194));
#14123=CARTESIAN_POINT('Origin',(-6.5,6.43177298256785,462.946209595194));
#14124=CARTESIAN_POINT('Origin',(-6.5,6.43177298256785,476.446209595194));
#14125=CARTESIAN_POINT('',(-15.5,6.43177298256785,463.346209595194));
#14126=CARTESIAN_POINT('',(-15.5,6.43177298256785,462.946209595194));
#14127=CARTESIAN_POINT('Origin',(-6.5,6.43177298256785,463.346209595194));
#14128=CARTESIAN_POINT('Origin',(-0.499999999999998,-0.276430949931514,
478.946209595194));
#14129=CARTESIAN_POINT('',(-0.499999999999999,10.4317729825678,471.090577685893));
#14130=CARTESIAN_POINT('Origin',(-0.499999999999999,6.43177298256785,471.090577685893));
#14131=CARTESIAN_POINT('Origin',(1.,6.43177298256785,464.946209595194));
#14132=CARTESIAN_POINT('Origin',(-6.5,6.43177298256785,476.446209595194));
#14133=CARTESIAN_POINT('Origin',(-6.5,6.43177298256785,463.346209595194));
#14134=CARTESIAN_POINT('',(-15.1,6.43177298256785,462.946209595194));
#14135=CARTESIAN_POINT('Origin',(-15.1,6.43177298256785,463.346209595194));
#14136=CARTESIAN_POINT('Origin',(-6.5,6.43177298256785,462.946209595194));
#14137=CARTESIAN_POINT('Origin',(-6.5,6.43177298256785,462.946209595194));
#14138=CARTESIAN_POINT('',(-13.9,6.43177298256785,462.946209595194));
#14139=CARTESIAN_POINT('Origin',(-6.5,6.43177298256785,462.946209595194));
#14140=CARTESIAN_POINT('Origin',(-6.5,6.43177298256785,462.546209595194));
#14141=CARTESIAN_POINT('',(-13.5,6.43177298256785,462.546209595194));
#14142=CARTESIAN_POINT('Origin',(-6.5,6.43177298256785,462.546209595194));
#14143=CARTESIAN_POINT('Origin',(-13.9,6.43177298256785,462.546209595194));
#14144=CARTESIAN_POINT('Origin',(-6.5,6.43177298256785,462.946209595194));
#14145=CARTESIAN_POINT('',(-13.5,6.43177298256785,451.346209595194));
#14146=CARTESIAN_POINT('',(0.499999999999999,6.43177298256785,451.346209595194));
#14147=CARTESIAN_POINT('Origin',(-6.5,6.43177298256785,451.346209595194));
#14148=CARTESIAN_POINT('',(-13.5,6.43177298256785,462.946209595194));
#14149=CARTESIAN_POINT('Origin',(-6.5,6.43177298256785,451.346209595194));
#14150=CARTESIAN_POINT('Origin',(-6.5,6.43177298256785,451.346209595194));
#14151=CARTESIAN_POINT('',(0.099999999999999,6.43177298256785,450.946209595194));
#14152=CARTESIAN_POINT('Origin',(-6.5,6.43177298256785,450.946209595194));
#14153=CARTESIAN_POINT('Origin',(0.099999999999999,6.43177298256785,451.346209595194));
#14154=CARTESIAN_POINT('Origin',(-6.5,6.43177298256785,450.946209595194));
#14155=CARTESIAN_POINT('',(-12.5,6.43177298256785,450.946209595194));
#14156=CARTESIAN_POINT('Origin',(-6.5,6.43177298256785,450.946209595194));
#14157=CARTESIAN_POINT('Origin',(-6.5,6.43177298256785,451.446209595194));
#14158=CARTESIAN_POINT('',(-11.5,6.43177298256785,451.946209595194));
#14159=CARTESIAN_POINT('',(-12.,6.43177298256785,451.446209595194));
#14160=CARTESIAN_POINT('Origin',(-6.5,6.43177298256785,451.946209595194));
#14161=CARTESIAN_POINT('Origin',(-6.5,6.43177298256785,462.946209595194));
#14162=CARTESIAN_POINT('',(-11.5,6.43177298256785,462.946209595194));
#14163=CARTESIAN_POINT('',(-11.5,6.43177298256785,462.946209595194));
#14164=CARTESIAN_POINT('Origin',(-6.5,6.43177298256785,462.946209595194));
#14165=CARTESIAN_POINT('Origin',(-12.5,6.43177298256785,471.090577685893));
#14166=CARTESIAN_POINT('',(-12.5,10.4317729825678,471.090577685893));
#14167=CARTESIAN_POINT('Origin',(-6.5,6.43177298256785,462.946209595194));
#17021=UNCERTAINTY_MEASURE_WITH_UNIT(LENGTH_MEASURE(0.01),#17043,
'DISTANCE_ACCURACY_VALUE',
'Maximum model space distance between geometric entities at asserted c
onnectivities');
#17028=UNCERTAINTY_MEASURE_WITH_UNIT(LENGTH_MEASURE(0.01),#17043,
'DISTANCE_ACCURACY_VALUE',
'Maximum model space distance between geometric entities at asserted c
onnectivities');
#17035=(
GEOMETRIC_REPRESENTATION_CONTEXT(3)
GLOBAL_UNCERTAINTY_ASSIGNED_CONTEXT((#17021))
GLOBAL_UNIT_ASSIGNED_CONTEXT((#17043,#17045,#17046))
REPRESENTATION_CONTEXT('','3D')
);
#17042=(
GEOMETRIC_REPRESENTATION_CONTEXT(3)
GLOBAL_UNCERTAINTY_ASSIGNED_CONTEXT((#17028))
GLOBAL_UNIT_ASSIGNED_CONTEXT((#17043,#17045,#17046))
REPRESENTATION_CONTEXT('','3D')
);
#17043=(
LENGTH_UNIT()
NAMED_UNIT(*)
SI_UNIT(.MILLI.,.METRE.)
);
#17045=(
NAMED_UNIT(*)
PLANE_ANGLE_UNIT()
SI_UNIT($,.RADIAN.)
);
#17046=(
NAMED_UNIT(*)
SI_UNIT($,.STERADIAN.)
SOLID_ANGLE_UNIT()
);
#17053=SHAPE_DEFINITION_REPRESENTATION(#17066,#17091);
#17066=PRODUCT_DEFINITION_SHAPE('',$,#17105);
#17091=SHAPE_REPRESENTATION('',(#8839),#17035);
#17098=PRODUCT_DEFINITION_CONTEXT('part definition',#17139,'design');
#17105=PRODUCT_DEFINITION('PLUG','PLUG',#17118,#17098);
#17118=PRODUCT_DEFINITION_FORMATION('',$,#17147);
#17139=APPLICATION_CONTEXT(
'Core Data for Automotive Mechanical Design Process');
#17140=PRODUCT_CONTEXT('part definition',#17139,'mechanical');
#17147=PRODUCT('PLUG','PLUG',$,(#17140));
#17154=PRESENTATION_STYLE_ASSIGNMENT((#17155));
#17155=SURFACE_STYLE_USAGE(.BOTH.,#17156);
#17156=SURFACE_SIDE_STYLE('',(#17157));
#17157=SURFACE_STYLE_FILL_AREA(#17158);
#17158=FILL_AREA_STYLE('Steel - Satin',(#17159));
#17159=FILL_AREA_STYLE_COLOUR('Steel - Satin',#17160);
#17160=COLOUR_RGB('Steel - Satin', 0.09019608, 0.27058824, 0.51372549);
ENDSEC;
END-ISO-10303-21;
